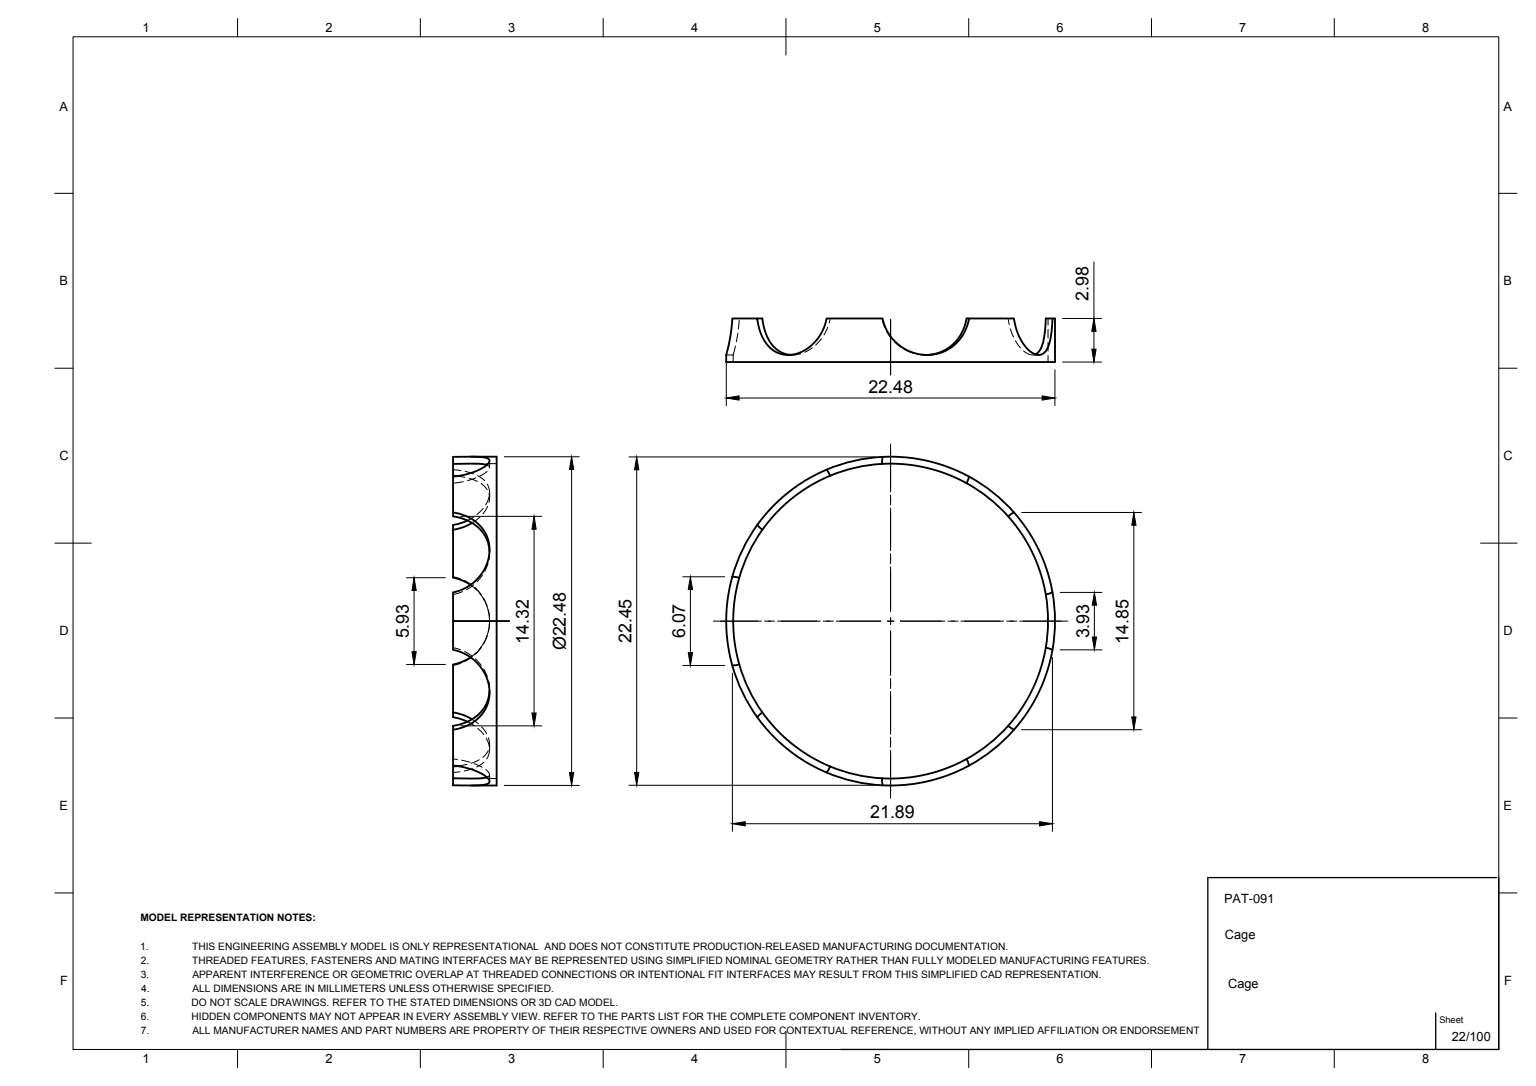
ISO-10303-21;
HEADER;
/* Generated by software containing ST-Developer
 * from STEP Tools, Inc. (www.steptools.com) 
 */

FILE_DESCRIPTION(
/* description */ ('PAT-091'),
/* implementation_level */ '2;1');

FILE_NAME(
/* name */ 'Cage.step',
/* time_stamp */ '2026-10-27T15:34:44-07:00',
/* author */ (''),
/* organization */ (''),
/* preprocessor_version */ 'ST-DEVELOPER v20.2',
/* originating_system */ 'Autodesk Translation Framework v15.17.0.0',
/* authorisation */ '');

FILE_SCHEMA (('AUTOMOTIVE_DESIGN { 1 0 10303 214 3 1 1 }'));
ENDSEC;

DATA;
#10=MECHANICAL_DESIGN_GEOMETRIC_PRESENTATION_REPRESENTATION('',(#1079,#1080,#1081,#1082,#1083,#1084,#1085),#25100);
#21=SPHERICAL_SURFACE('',#16189,0.321462);
#22=SPHERICAL_SURFACE('',#16202,0.321462);
#23=SPHERICAL_SURFACE('',#16203,0.321462);
#24=SPHERICAL_SURFACE('',#16216,0.321462);
#25=SPHERICAL_SURFACE('',#16217,0.321462);
#26=SPHERICAL_SURFACE('',#16230,0.321462);
#27=SPHERICAL_SURFACE('',#16231,0.321462);
#28=SPHERICAL_SURFACE('',#16244,0.321462);
#29=SPHERICAL_SURFACE('',#16245,0.321462);
#30=SPHERICAL_SURFACE('',#16258,0.321462);
#31=SPHERICAL_SURFACE('',#16259,0.321462);
#32=SPHERICAL_SURFACE('',#16272,0.321462);
#33=SPHERICAL_SURFACE('',#16280,0.321462);
#34=SPHERICAL_SURFACE('',#16286,0.321462);
#701=B_SPLINE_CURVE_WITH_KNOTS('',3,(#24299,#24300,#24301,#24302,#24303,
#24304),.UNSPECIFIED.,.F.,.F.,(4,2,4),(0.899240844561108,0.954818878854282,
0.98574345825674),.UNSPECIFIED.);
#702=B_SPLINE_CURVE_WITH_KNOTS('',3,(#24308,#24309,#24310,#24311,#24312,
#24313),.UNSPECIFIED.,.F.,.F.,(4,2,4),(1.23862523261148,1.28156721462942,
1.33421556357425),.UNSPECIFIED.);
#703=B_SPLINE_CURVE_WITH_KNOTS('',3,(#24324,#24325,#24326,#24327,#24328,
#24329),.UNSPECIFIED.,.F.,.F.,(4,2,4),(0.959827414101938,1.01247576304677,
1.05541774506471),.UNSPECIFIED.);
#704=B_SPLINE_CURVE_WITH_KNOTS('',3,(#24335,#24336,#24337,#24338,#24339,
#24340),.UNSPECIFIED.,.F.,.F.,(4,2,4),(1.13866312806976,1.16958770747221,
1.22516574176539),.UNSPECIFIED.);
#705=B_SPLINE_CURVE_WITH_KNOTS('',3,(#24347,#24348,#24349,#24350,#24351,
#24352),.UNSPECIFIED.,.F.,.F.,(4,2,4),(0.899240844561108,0.954818878854283,
0.985743458256741),.UNSPECIFIED.);
#706=B_SPLINE_CURVE_WITH_KNOTS('',3,(#24355,#24356,#24357,#24358,#24359,
#24360),.UNSPECIFIED.,.F.,.F.,(4,2,4),(1.23862523261148,1.28156721462942,
1.33421556357425),.UNSPECIFIED.);
#707=B_SPLINE_CURVE_WITH_KNOTS('',3,(#24369,#24370,#24371,#24372,#24373,
#24374),.UNSPECIFIED.,.F.,.F.,(4,2,4),(0.959827414101939,1.01247576304677,
1.05541774506471),.UNSPECIFIED.);
#708=B_SPLINE_CURVE_WITH_KNOTS('',3,(#24379,#24380,#24381,#24382,#24383,
#24384),.UNSPECIFIED.,.F.,.F.,(4,2,4),(1.13866312806975,1.16958770747221,
1.22516574176539),.UNSPECIFIED.);
#709=B_SPLINE_CURVE_WITH_KNOTS('',3,(#24391,#24392,#24393,#24394,#24395,
#24396),.UNSPECIFIED.,.F.,.F.,(4,2,4),(0.899240844561107,0.954818878854282,
0.98574345825674),.UNSPECIFIED.);
#710=B_SPLINE_CURVE_WITH_KNOTS('',3,(#24400,#24401,#24402,#24403,#24404,
#24405),.UNSPECIFIED.,.F.,.F.,(4,2,4),(1.23862523261148,1.28156721462942,
1.33421556357425),.UNSPECIFIED.);
#711=B_SPLINE_CURVE_WITH_KNOTS('',3,(#24411,#24412,#24413,#24414,#24415,
#24416),.UNSPECIFIED.,.F.,.F.,(4,2,4),(0.959827414101938,1.01247576304677,
1.05541774506471),.UNSPECIFIED.);
#712=B_SPLINE_CURVE_WITH_KNOTS('',3,(#24427,#24428,#24429,#24430,#24431,
#24432),.UNSPECIFIED.,.F.,.F.,(4,2,4),(1.13866312806976,1.16958770747221,
1.22516574176539),.UNSPECIFIED.);
#713=B_SPLINE_CURVE_WITH_KNOTS('',3,(#24439,#24440,#24441,#24442,#24443,
#24444),.UNSPECIFIED.,.F.,.F.,(4,2,4),(1.13866312806976,1.16958770747221,
1.22516574176539),.UNSPECIFIED.);
#714=B_SPLINE_CURVE_WITH_KNOTS('',3,(#24447,#24448,#24449,#24450,#24451,
#24452),.UNSPECIFIED.,.F.,.F.,(4,2,4),(0.959827414101938,1.01247576304677,
1.05541774506471),.UNSPECIFIED.);
#715=B_SPLINE_CURVE_WITH_KNOTS('',3,(#24457,#24458,#24459,#24460,#24461,
#24462),.UNSPECIFIED.,.F.,.F.,(4,2,4),(1.23862523261148,1.28156721462942,
1.33421556357425),.UNSPECIFIED.);
#716=B_SPLINE_CURVE_WITH_KNOTS('',3,(#24471,#24472,#24473,#24474,#24475,
#24476),.UNSPECIFIED.,.F.,.F.,(4,2,4),(0.899240844561108,0.954818878854282,
0.985743458256741),.UNSPECIFIED.);
#717=B_SPLINE_CURVE_WITH_KNOTS('',3,(#24483,#24484,#24485,#24486,#24487,
#24488),.UNSPECIFIED.,.F.,.F.,(4,2,4),(1.13866312806975,1.16958770747221,
1.22516574176539),.UNSPECIFIED.);
#718=B_SPLINE_CURVE_WITH_KNOTS('',3,(#24492,#24493,#24494,#24495,#24496,
#24497),.UNSPECIFIED.,.F.,.F.,(4,2,4),(0.959827414101939,1.01247576304677,
1.05541774506471),.UNSPECIFIED.);
#719=B_SPLINE_CURVE_WITH_KNOTS('',3,(#24502,#24503,#24504,#24505,#24506,
#24507),.UNSPECIFIED.,.F.,.F.,(4,2,4),(0.899240844561108,0.954818878854282,
0.985743458256741),.UNSPECIFIED.);
#720=B_SPLINE_CURVE_WITH_KNOTS('',3,(#24519,#24520,#24521,#24522,#24523,
#24524),.UNSPECIFIED.,.F.,.F.,(4,2,4),(1.23862523261148,1.28156721462942,
1.33421556357425),.UNSPECIFIED.);
#721=B_SPLINE_CURVE_WITH_KNOTS('',3,(#24529,#24530,#24531,#24532,#24533,
#24534),.UNSPECIFIED.,.F.,.F.,(4,2,4),(1.13866312806976,1.16958770747221,
1.22516574176539),.UNSPECIFIED.);
#722=B_SPLINE_CURVE_WITH_KNOTS('',3,(#24538,#24539,#24540,#24541,#24542,
#24543),.UNSPECIFIED.,.F.,.F.,(4,2,4),(0.959827414101938,1.01247576304677,
1.05541774506471),.UNSPECIFIED.);
#723=B_SPLINE_CURVE_WITH_KNOTS('',3,(#24548,#24549,#24550,#24551,#24552,
#24553),.UNSPECIFIED.,.F.,.F.,(4,2,4),(0.899240844561108,0.954818878854282,
0.98574345825674),.UNSPECIFIED.);
#724=B_SPLINE_CURVE_WITH_KNOTS('',3,(#24562,#24563,#24564,#24565,#24566,
#24567),.UNSPECIFIED.,.F.,.F.,(4,2,4),(1.23862523261148,1.28156721462942,
1.33421556357425),.UNSPECIFIED.);
#725=B_SPLINE_CURVE_WITH_KNOTS('',3,(#24575,#24576,#24577,#24578,#24579,
#24580),.UNSPECIFIED.,.F.,.F.,(4,2,4),(1.23862523261148,1.28156721462942,
1.33421556357425),.UNSPECIFIED.);
#726=B_SPLINE_CURVE_WITH_KNOTS('',3,(#24584,#24585,#24586,#24587,#24588,
#24589),.UNSPECIFIED.,.F.,.F.,(4,2,4),(0.959827414101938,1.01247576304677,
1.05541774506471),.UNSPECIFIED.);
#727=B_SPLINE_CURVE_WITH_KNOTS('',3,(#24600,#24601,#24602,#24603,#24604,
#24605),.UNSPECIFIED.,.F.,.F.,(4,2,4),(1.13866312806976,1.16958770747221,
1.22516574176539),.UNSPECIFIED.);
#728=B_SPLINE_CURVE_WITH_KNOTS('',3,(#24611,#24612,#24613,#24614,#24615,
#24616),.UNSPECIFIED.,.F.,.F.,(4,2,4),(0.899240844561108,0.954818878854282,
0.98574345825674),.UNSPECIFIED.);
#853=SHAPE_REPRESENTATION_RELATIONSHIP('SRR','None',#25621,#963);
#963=ADVANCED_BREP_SHAPE_REPRESENTATION('',(#1200,#1201,#1202,#1203,#1204,
#1205,#1206),#25091);
#1079=STYLED_ITEM('',(#26191),#1200);
#1080=STYLED_ITEM('',(#26191),#1201);
#1081=STYLED_ITEM('',(#26191),#1202);
#1082=STYLED_ITEM('',(#26191),#1203);
#1083=STYLED_ITEM('',(#26191),#1204);
#1084=STYLED_ITEM('',(#26191),#1205);
#1085=STYLED_ITEM('',(#26191),#1206);
#1200=MANIFOLD_SOLID_BREP('Body1',#13359);
#1201=MANIFOLD_SOLID_BREP('Body9',#13360);
#1202=MANIFOLD_SOLID_BREP('Body10',#13361);
#1203=MANIFOLD_SOLID_BREP('Body11',#13362);
#1204=MANIFOLD_SOLID_BREP('Body12',#13363);
#1205=MANIFOLD_SOLID_BREP('Body13',#13364);
#1206=MANIFOLD_SOLID_BREP('Body14',#13365);
#2028=PLANE('',#16192);
#2029=PLANE('',#16198);
#2030=PLANE('',#16206);
#2031=PLANE('',#16214);
#2032=PLANE('',#16223);
#2033=PLANE('',#16226);
#2034=PLANE('',#16237);
#2035=PLANE('',#16242);
#2036=PLANE('',#16251);
#2037=PLANE('',#16254);
#2038=PLANE('',#16265);
#2039=PLANE('',#16270);
#2040=PLANE('',#16276);
#2041=PLANE('',#16282);
#2798=FACE_OUTER_BOUND('',#4022,.T.);
#2799=FACE_OUTER_BOUND('',#4023,.T.);
#2800=FACE_OUTER_BOUND('',#4024,.T.);
#2801=FACE_OUTER_BOUND('',#4025,.T.);
#2802=FACE_OUTER_BOUND('',#4026,.T.);
#2803=FACE_OUTER_BOUND('',#4027,.T.);
#2804=FACE_OUTER_BOUND('',#4028,.T.);
#2805=FACE_OUTER_BOUND('',#4029,.T.);
#2806=FACE_OUTER_BOUND('',#4030,.T.);
#2807=FACE_OUTER_BOUND('',#4031,.T.);
#2808=FACE_OUTER_BOUND('',#4032,.T.);
#2809=FACE_OUTER_BOUND('',#4033,.T.);
#2810=FACE_OUTER_BOUND('',#4034,.T.);
#2811=FACE_OUTER_BOUND('',#4035,.T.);
#2812=FACE_OUTER_BOUND('',#4036,.T.);
#2813=FACE_OUTER_BOUND('',#4037,.T.);
#2814=FACE_OUTER_BOUND('',#4038,.T.);
#2815=FACE_OUTER_BOUND('',#4039,.T.);
#2816=FACE_OUTER_BOUND('',#4040,.T.);
#2817=FACE_OUTER_BOUND('',#4041,.T.);
#2818=FACE_OUTER_BOUND('',#4042,.T.);
#2819=FACE_OUTER_BOUND('',#4043,.T.);
#2820=FACE_OUTER_BOUND('',#4044,.T.);
#2821=FACE_OUTER_BOUND('',#4045,.T.);
#2822=FACE_OUTER_BOUND('',#4046,.T.);
#2823=FACE_OUTER_BOUND('',#4047,.T.);
#2824=FACE_OUTER_BOUND('',#4048,.T.);
#2825=FACE_OUTER_BOUND('',#4049,.T.);
#2826=FACE_OUTER_BOUND('',#4050,.T.);
#2827=FACE_OUTER_BOUND('',#4051,.T.);
#2828=FACE_OUTER_BOUND('',#4052,.T.);
#2829=FACE_OUTER_BOUND('',#4053,.T.);
#2830=FACE_OUTER_BOUND('',#4054,.T.);
#2831=FACE_OUTER_BOUND('',#4055,.T.);
#2832=FACE_OUTER_BOUND('',#4056,.T.);
#2833=FACE_OUTER_BOUND('',#4057,.T.);
#2834=FACE_OUTER_BOUND('',#4058,.T.);
#2835=FACE_OUTER_BOUND('',#4059,.T.);
#2836=FACE_OUTER_BOUND('',#4060,.T.);
#2837=FACE_OUTER_BOUND('',#4061,.T.);
#2838=FACE_OUTER_BOUND('',#4062,.T.);
#2839=FACE_OUTER_BOUND('',#4063,.T.);
#4022=EDGE_LOOP('',(#11786,#11787,#11788,#11789));
#4023=EDGE_LOOP('',(#11790,#11791,#11792,#11793));
#4024=EDGE_LOOP('',(#11794,#11795,#11796,#11797));
#4025=EDGE_LOOP('',(#11798,#11799,#11800,#11801));
#4026=EDGE_LOOP('',(#11802,#11803,#11804,#11805));
#4027=EDGE_LOOP('',(#11806,#11807,#11808,#11809));
#4028=EDGE_LOOP('',(#11810,#11811,#11812,#11813));
#4029=EDGE_LOOP('',(#11814,#11815,#11816,#11817));
#4030=EDGE_LOOP('',(#11818,#11819,#11820,#11821));
#4031=EDGE_LOOP('',(#11822,#11823,#11824,#11825));
#4032=EDGE_LOOP('',(#11826,#11827,#11828,#11829));
#4033=EDGE_LOOP('',(#11830,#11831,#11832,#11833));
#4034=EDGE_LOOP('',(#11834,#11835,#11836,#11837));
#4035=EDGE_LOOP('',(#11838,#11839,#11840,#11841));
#4036=EDGE_LOOP('',(#11842,#11843,#11844,#11845));
#4037=EDGE_LOOP('',(#11846,#11847,#11848,#11849));
#4038=EDGE_LOOP('',(#11850,#11851,#11852,#11853));
#4039=EDGE_LOOP('',(#11854,#11855,#11856,#11857));
#4040=EDGE_LOOP('',(#11858,#11859,#11860,#11861));
#4041=EDGE_LOOP('',(#11862,#11863,#11864,#11865));
#4042=EDGE_LOOP('',(#11866,#11867,#11868,#11869));
#4043=EDGE_LOOP('',(#11870,#11871,#11872,#11873));
#4044=EDGE_LOOP('',(#11874,#11875,#11876,#11877));
#4045=EDGE_LOOP('',(#11878,#11879,#11880,#11881));
#4046=EDGE_LOOP('',(#11882,#11883,#11884,#11885));
#4047=EDGE_LOOP('',(#11886,#11887,#11888,#11889));
#4048=EDGE_LOOP('',(#11890,#11891,#11892,#11893));
#4049=EDGE_LOOP('',(#11894,#11895,#11896,#11897));
#4050=EDGE_LOOP('',(#11898,#11899,#11900,#11901));
#4051=EDGE_LOOP('',(#11902,#11903,#11904,#11905));
#4052=EDGE_LOOP('',(#11906,#11907,#11908,#11909));
#4053=EDGE_LOOP('',(#11910,#11911,#11912,#11913));
#4054=EDGE_LOOP('',(#11914,#11915,#11916,#11917));
#4055=EDGE_LOOP('',(#11918,#11919,#11920,#11921));
#4056=EDGE_LOOP('',(#11922,#11923,#11924,#11925));
#4057=EDGE_LOOP('',(#11926,#11927,#11928,#11929));
#4058=EDGE_LOOP('',(#11930,#11931,#11932,#11933));
#4059=EDGE_LOOP('',(#11934,#11935,#11936,#11937));
#4060=EDGE_LOOP('',(#11938,#11939,#11940,#11941));
#4061=EDGE_LOOP('',(#11942,#11943,#11944,#11945));
#4062=EDGE_LOOP('',(#11946,#11947,#11948,#11949));
#4063=EDGE_LOOP('',(#11950,#11951,#11952,#11953));
#6287=CIRCLE('',#16190,0.267289037081583);
#6288=CIRCLE('',#16191,0.226018648221778);
#6289=CIRCLE('',#16193,1.308355);
#6290=CIRCLE('',#16194,0.226018648221778);
#6291=CIRCLE('',#16195,0.891645);
#6292=CIRCLE('',#16197,1.308355);
#6293=CIRCLE('',#16199,0.891645);
#6294=CIRCLE('',#16200,0.267289037081583);
#6295=CIRCLE('',#16204,0.226018648221778);
#6296=CIRCLE('',#16205,0.267289037081583);
#6297=CIRCLE('',#16207,0.891645);
#6298=CIRCLE('',#16208,0.267289037081583);
#6299=CIRCLE('',#16209,1.308355);
#6300=CIRCLE('',#16211,1.308355);
#6301=CIRCLE('',#16213,0.891645);
#6302=CIRCLE('',#16215,0.226018648221778);
#6303=CIRCLE('',#16218,0.267289037081583);
#6304=CIRCLE('',#16219,0.226018648221778);
#6305=CIRCLE('',#16221,1.308355);
#6306=CIRCLE('',#16222,1.308355);
#6307=CIRCLE('',#16224,0.226018648221778);
#6308=CIRCLE('',#16225,0.891645);
#6309=CIRCLE('',#16227,0.891645);
#6310=CIRCLE('',#16228,0.267289037081583);
#6311=CIRCLE('',#16232,0.267289037081583);
#6312=CIRCLE('',#16233,0.226018648221778);
#6313=CIRCLE('',#16235,1.308355);
#6314=CIRCLE('',#16236,1.308355);
#6315=CIRCLE('',#16238,0.891645);
#6316=CIRCLE('',#16239,0.226018648221778);
#6317=CIRCLE('',#16241,0.891645);
#6318=CIRCLE('',#16243,0.267289037081583);
#6319=CIRCLE('',#16246,0.226018648221778);
#6320=CIRCLE('',#16247,0.267289037081583);
#6321=CIRCLE('',#16249,0.891645);
#6322=CIRCLE('',#16250,0.891645);
#6323=CIRCLE('',#16252,0.267289037081583);
#6324=CIRCLE('',#16253,1.308355);
#6325=CIRCLE('',#16255,0.226018648221778);
#6326=CIRCLE('',#16256,1.308355);
#6327=CIRCLE('',#16260,0.226018648221778);
#6328=CIRCLE('',#16261,0.267289037081583);
#6329=CIRCLE('',#16263,0.891645);
#6330=CIRCLE('',#16264,0.891645);
#6331=CIRCLE('',#16266,0.267289037081583);
#6332=CIRCLE('',#16267,1.308355);
#6333=CIRCLE('',#16269,1.308355);
#6334=CIRCLE('',#16271,0.226018648221778);
#6335=CIRCLE('',#16274,1.308355);
#6336=CIRCLE('',#16275,1.308355);
#6337=CIRCLE('',#16277,0.226018648221778);
#6338=CIRCLE('',#16278,0.226018648221778);
#6339=CIRCLE('',#16279,0.891645);
#6340=CIRCLE('',#16281,0.267289037081583);
#6341=CIRCLE('',#16283,0.267289037081583);
#6342=CIRCLE('',#16284,0.891645);
#7325=VERTEX_POINT('',#24297);
#7326=VERTEX_POINT('',#24298);
#7327=VERTEX_POINT('',#24305);
#7328=VERTEX_POINT('',#24307);
#7329=VERTEX_POINT('',#24316);
#7330=VERTEX_POINT('',#24318);
#7331=VERTEX_POINT('',#24322);
#7332=VERTEX_POINT('',#24331);
#7333=VERTEX_POINT('',#24343);
#7334=VERTEX_POINT('',#24344);
#7335=VERTEX_POINT('',#24346);
#7336=VERTEX_POINT('',#24353);
#7337=VERTEX_POINT('',#24362);
#7338=VERTEX_POINT('',#24364);
#7339=VERTEX_POINT('',#24368);
#7340=VERTEX_POINT('',#24377);
#7341=VERTEX_POINT('',#24389);
#7342=VERTEX_POINT('',#24390);
#7343=VERTEX_POINT('',#24397);
#7344=VERTEX_POINT('',#24399);
#7345=VERTEX_POINT('',#24408);
#7346=VERTEX_POINT('',#24410);
#7347=VERTEX_POINT('',#24419);
#7348=VERTEX_POINT('',#24423);
#7349=VERTEX_POINT('',#24435);
#7350=VERTEX_POINT('',#24436);
#7351=VERTEX_POINT('',#24438);
#7352=VERTEX_POINT('',#24445);
#7353=VERTEX_POINT('',#24454);
#7354=VERTEX_POINT('',#24456);
#7355=VERTEX_POINT('',#24465);
#7356=VERTEX_POINT('',#24469);
#7357=VERTEX_POINT('',#24481);
#7358=VERTEX_POINT('',#24482);
#7359=VERTEX_POINT('',#24489);
#7360=VERTEX_POINT('',#24491);
#7361=VERTEX_POINT('',#24500);
#7362=VERTEX_POINT('',#24501);
#7363=VERTEX_POINT('',#24511);
#7364=VERTEX_POINT('',#24515);
#7365=VERTEX_POINT('',#24527);
#7366=VERTEX_POINT('',#24528);
#7367=VERTEX_POINT('',#24535);
#7368=VERTEX_POINT('',#24537);
#7369=VERTEX_POINT('',#24546);
#7370=VERTEX_POINT('',#24547);
#7371=VERTEX_POINT('',#24557);
#7372=VERTEX_POINT('',#24561);
#7373=VERTEX_POINT('',#24573);
#7374=VERTEX_POINT('',#24574);
#7375=VERTEX_POINT('',#24581);
#7376=VERTEX_POINT('',#24583);
#7377=VERTEX_POINT('',#24592);
#7378=VERTEX_POINT('',#24594);
#7379=VERTEX_POINT('',#24598);
#7380=VERTEX_POINT('',#24607);
#8828=EDGE_CURVE('',#7325,#7326,#701,.T.);
#8829=EDGE_CURVE('',#7327,#7325,#6287,.T.);
#8830=EDGE_CURVE('',#7328,#7327,#702,.T.);
#8831=EDGE_CURVE('',#7326,#7328,#6288,.T.);
#8832=EDGE_CURVE('',#7328,#7329,#6289,.T.);
#8833=EDGE_CURVE('',#7329,#7330,#6290,.T.);
#8834=EDGE_CURVE('',#7326,#7330,#6291,.T.);
#8835=EDGE_CURVE('',#7327,#7331,#6292,.T.);
#8836=EDGE_CURVE('',#7331,#7329,#703,.T.);
#8837=EDGE_CURVE('',#7325,#7332,#6293,.T.);
#8838=EDGE_CURVE('',#7332,#7331,#6294,.T.);
#8839=EDGE_CURVE('',#7330,#7332,#704,.T.);
#8840=EDGE_CURVE('',#7333,#7334,#6295,.T.);
#8841=EDGE_CURVE('',#7335,#7333,#705,.T.);
#8842=EDGE_CURVE('',#7336,#7335,#6296,.T.);
#8843=EDGE_CURVE('',#7334,#7336,#706,.T.);
#8844=EDGE_CURVE('',#7335,#7337,#6297,.T.);
#8845=EDGE_CURVE('',#7337,#7338,#6298,.T.);
#8846=EDGE_CURVE('',#7336,#7338,#6299,.T.);
#8847=EDGE_CURVE('',#7338,#7339,#707,.T.);
#8848=EDGE_CURVE('',#7334,#7339,#6300,.T.);
#8849=EDGE_CURVE('',#7333,#7340,#6301,.T.);
#8850=EDGE_CURVE('',#7340,#7337,#708,.T.);
#8851=EDGE_CURVE('',#7339,#7340,#6302,.T.);
#8852=EDGE_CURVE('',#7341,#7342,#709,.T.);
#8853=EDGE_CURVE('',#7343,#7341,#6303,.T.);
#8854=EDGE_CURVE('',#7344,#7343,#710,.T.);
#8855=EDGE_CURVE('',#7342,#7344,#6304,.T.);
#8856=EDGE_CURVE('',#7343,#7345,#6305,.T.);
#8857=EDGE_CURVE('',#7345,#7346,#711,.T.);
#8858=EDGE_CURVE('',#7344,#7346,#6306,.T.);
#8859=EDGE_CURVE('',#7346,#7347,#6307,.T.);
#8860=EDGE_CURVE('',#7342,#7347,#6308,.T.);
#8861=EDGE_CURVE('',#7341,#7348,#6309,.T.);
#8862=EDGE_CURVE('',#7348,#7345,#6310,.T.);
#8863=EDGE_CURVE('',#7347,#7348,#712,.T.);
#8864=EDGE_CURVE('',#7349,#7350,#6311,.T.);
#8865=EDGE_CURVE('',#7351,#7349,#713,.T.);
#8866=EDGE_CURVE('',#7352,#7351,#6312,.T.);
#8867=EDGE_CURVE('',#7350,#7352,#714,.T.);
#8868=EDGE_CURVE('',#7353,#7352,#6313,.T.);
#8869=EDGE_CURVE('',#7353,#7354,#715,.T.);
#8870=EDGE_CURVE('',#7354,#7350,#6314,.T.);
#8871=EDGE_CURVE('',#7355,#7351,#6315,.T.);
#8872=EDGE_CURVE('',#7355,#7353,#6316,.T.);
#8873=EDGE_CURVE('',#7356,#7349,#6317,.T.);
#8874=EDGE_CURVE('',#7356,#7355,#716,.T.);
#8875=EDGE_CURVE('',#7354,#7356,#6318,.T.);
#8876=EDGE_CURVE('',#7357,#7358,#717,.T.);
#8877=EDGE_CURVE('',#7359,#7357,#6319,.T.);
#8878=EDGE_CURVE('',#7360,#7359,#718,.T.);
#8879=EDGE_CURVE('',#7358,#7360,#6320,.T.);
#8880=EDGE_CURVE('',#7361,#7362,#719,.T.);
#8881=EDGE_CURVE('',#7362,#7357,#6321,.T.);
#8882=EDGE_CURVE('',#7361,#7358,#6322,.T.);
#8883=EDGE_CURVE('',#7363,#7361,#6323,.T.);
#8884=EDGE_CURVE('',#7363,#7360,#6324,.T.);
#8885=EDGE_CURVE('',#7362,#7364,#6325,.T.);
#8886=EDGE_CURVE('',#7364,#7359,#6326,.T.);
#8887=EDGE_CURVE('',#7364,#7363,#720,.T.);
#8888=EDGE_CURVE('',#7365,#7366,#721,.T.);
#8889=EDGE_CURVE('',#7367,#7365,#6327,.T.);
#8890=EDGE_CURVE('',#7368,#7367,#722,.T.);
#8891=EDGE_CURVE('',#7366,#7368,#6328,.T.);
#8892=EDGE_CURVE('',#7369,#7370,#723,.T.);
#8893=EDGE_CURVE('',#7370,#7365,#6329,.T.);
#8894=EDGE_CURVE('',#7369,#7366,#6330,.T.);
#8895=EDGE_CURVE('',#7371,#7369,#6331,.T.);
#8896=EDGE_CURVE('',#7371,#7368,#6332,.T.);
#8897=EDGE_CURVE('',#7372,#7371,#724,.T.);
#8898=EDGE_CURVE('',#7372,#7367,#6333,.T.);
#8899=EDGE_CURVE('',#7370,#7372,#6334,.T.);
#8900=EDGE_CURVE('',#7373,#7374,#725,.T.);
#8901=EDGE_CURVE('',#7374,#7375,#6335,.T.);
#8902=EDGE_CURVE('',#7375,#7376,#726,.T.);
#8903=EDGE_CURVE('',#7373,#7376,#6336,.T.);
#8904=EDGE_CURVE('',#7377,#7373,#6337,.T.);
#8905=EDGE_CURVE('',#7376,#7378,#6338,.T.);
#8906=EDGE_CURVE('',#7377,#7378,#6339,.T.);
#8907=EDGE_CURVE('',#7379,#7375,#6340,.T.);
#8908=EDGE_CURVE('',#7378,#7379,#727,.T.);
#8909=EDGE_CURVE('',#7374,#7380,#6341,.T.);
#8910=EDGE_CURVE('',#7380,#7379,#6342,.T.);
#8911=EDGE_CURVE('',#7380,#7377,#728,.T.);
#11786=ORIENTED_EDGE('',*,*,#8828,.F.);
#11787=ORIENTED_EDGE('',*,*,#8829,.F.);
#11788=ORIENTED_EDGE('',*,*,#8830,.F.);
#11789=ORIENTED_EDGE('',*,*,#8831,.F.);
#11790=ORIENTED_EDGE('',*,*,#8831,.T.);
#11791=ORIENTED_EDGE('',*,*,#8832,.T.);
#11792=ORIENTED_EDGE('',*,*,#8833,.T.);
#11793=ORIENTED_EDGE('',*,*,#8834,.F.);
#11794=ORIENTED_EDGE('',*,*,#8830,.T.);
#11795=ORIENTED_EDGE('',*,*,#8835,.T.);
#11796=ORIENTED_EDGE('',*,*,#8836,.T.);
#11797=ORIENTED_EDGE('',*,*,#8832,.F.);
#11798=ORIENTED_EDGE('',*,*,#8829,.T.);
#11799=ORIENTED_EDGE('',*,*,#8837,.T.);
#11800=ORIENTED_EDGE('',*,*,#8838,.T.);
#11801=ORIENTED_EDGE('',*,*,#8835,.F.);
#11802=ORIENTED_EDGE('',*,*,#8828,.T.);
#11803=ORIENTED_EDGE('',*,*,#8834,.T.);
#11804=ORIENTED_EDGE('',*,*,#8839,.T.);
#11805=ORIENTED_EDGE('',*,*,#8837,.F.);
#11806=ORIENTED_EDGE('',*,*,#8833,.F.);
#11807=ORIENTED_EDGE('',*,*,#8836,.F.);
#11808=ORIENTED_EDGE('',*,*,#8838,.F.);
#11809=ORIENTED_EDGE('',*,*,#8839,.F.);
#11810=ORIENTED_EDGE('',*,*,#8840,.F.);
#11811=ORIENTED_EDGE('',*,*,#8841,.F.);
#11812=ORIENTED_EDGE('',*,*,#8842,.F.);
#11813=ORIENTED_EDGE('',*,*,#8843,.F.);
#11814=ORIENTED_EDGE('',*,*,#8842,.T.);
#11815=ORIENTED_EDGE('',*,*,#8844,.T.);
#11816=ORIENTED_EDGE('',*,*,#8845,.T.);
#11817=ORIENTED_EDGE('',*,*,#8846,.F.);
#11818=ORIENTED_EDGE('',*,*,#8843,.T.);
#11819=ORIENTED_EDGE('',*,*,#8846,.T.);
#11820=ORIENTED_EDGE('',*,*,#8847,.T.);
#11821=ORIENTED_EDGE('',*,*,#8848,.F.);
#11822=ORIENTED_EDGE('',*,*,#8841,.T.);
#11823=ORIENTED_EDGE('',*,*,#8849,.T.);
#11824=ORIENTED_EDGE('',*,*,#8850,.T.);
#11825=ORIENTED_EDGE('',*,*,#8844,.F.);
#11826=ORIENTED_EDGE('',*,*,#8840,.T.);
#11827=ORIENTED_EDGE('',*,*,#8848,.T.);
#11828=ORIENTED_EDGE('',*,*,#8851,.T.);
#11829=ORIENTED_EDGE('',*,*,#8849,.F.);
#11830=ORIENTED_EDGE('',*,*,#8845,.F.);
#11831=ORIENTED_EDGE('',*,*,#8850,.F.);
#11832=ORIENTED_EDGE('',*,*,#8851,.F.);
#11833=ORIENTED_EDGE('',*,*,#8847,.F.);
#11834=ORIENTED_EDGE('',*,*,#8852,.F.);
#11835=ORIENTED_EDGE('',*,*,#8853,.F.);
#11836=ORIENTED_EDGE('',*,*,#8854,.F.);
#11837=ORIENTED_EDGE('',*,*,#8855,.F.);
#11838=ORIENTED_EDGE('',*,*,#8854,.T.);
#11839=ORIENTED_EDGE('',*,*,#8856,.T.);
#11840=ORIENTED_EDGE('',*,*,#8857,.T.);
#11841=ORIENTED_EDGE('',*,*,#8858,.F.);
#11842=ORIENTED_EDGE('',*,*,#8855,.T.);
#11843=ORIENTED_EDGE('',*,*,#8858,.T.);
#11844=ORIENTED_EDGE('',*,*,#8859,.T.);
#11845=ORIENTED_EDGE('',*,*,#8860,.F.);
#11846=ORIENTED_EDGE('',*,*,#8853,.T.);
#11847=ORIENTED_EDGE('',*,*,#8861,.T.);
#11848=ORIENTED_EDGE('',*,*,#8862,.T.);
#11849=ORIENTED_EDGE('',*,*,#8856,.F.);
#11850=ORIENTED_EDGE('',*,*,#8852,.T.);
#11851=ORIENTED_EDGE('',*,*,#8860,.T.);
#11852=ORIENTED_EDGE('',*,*,#8863,.T.);
#11853=ORIENTED_EDGE('',*,*,#8861,.F.);
#11854=ORIENTED_EDGE('',*,*,#8859,.F.);
#11855=ORIENTED_EDGE('',*,*,#8857,.F.);
#11856=ORIENTED_EDGE('',*,*,#8862,.F.);
#11857=ORIENTED_EDGE('',*,*,#8863,.F.);
#11858=ORIENTED_EDGE('',*,*,#8864,.F.);
#11859=ORIENTED_EDGE('',*,*,#8865,.F.);
#11860=ORIENTED_EDGE('',*,*,#8866,.F.);
#11861=ORIENTED_EDGE('',*,*,#8867,.F.);
#11862=ORIENTED_EDGE('',*,*,#8867,.T.);
#11863=ORIENTED_EDGE('',*,*,#8868,.F.);
#11864=ORIENTED_EDGE('',*,*,#8869,.T.);
#11865=ORIENTED_EDGE('',*,*,#8870,.T.);
#11866=ORIENTED_EDGE('',*,*,#8866,.T.);
#11867=ORIENTED_EDGE('',*,*,#8871,.F.);
#11868=ORIENTED_EDGE('',*,*,#8872,.T.);
#11869=ORIENTED_EDGE('',*,*,#8868,.T.);
#11870=ORIENTED_EDGE('',*,*,#8865,.T.);
#11871=ORIENTED_EDGE('',*,*,#8873,.F.);
#11872=ORIENTED_EDGE('',*,*,#8874,.T.);
#11873=ORIENTED_EDGE('',*,*,#8871,.T.);
#11874=ORIENTED_EDGE('',*,*,#8864,.T.);
#11875=ORIENTED_EDGE('',*,*,#8870,.F.);
#11876=ORIENTED_EDGE('',*,*,#8875,.T.);
#11877=ORIENTED_EDGE('',*,*,#8873,.T.);
#11878=ORIENTED_EDGE('',*,*,#8875,.F.);
#11879=ORIENTED_EDGE('',*,*,#8869,.F.);
#11880=ORIENTED_EDGE('',*,*,#8872,.F.);
#11881=ORIENTED_EDGE('',*,*,#8874,.F.);
#11882=ORIENTED_EDGE('',*,*,#8876,.F.);
#11883=ORIENTED_EDGE('',*,*,#8877,.F.);
#11884=ORIENTED_EDGE('',*,*,#8878,.F.);
#11885=ORIENTED_EDGE('',*,*,#8879,.F.);
#11886=ORIENTED_EDGE('',*,*,#8880,.T.);
#11887=ORIENTED_EDGE('',*,*,#8881,.T.);
#11888=ORIENTED_EDGE('',*,*,#8876,.T.);
#11889=ORIENTED_EDGE('',*,*,#8882,.F.);
#11890=ORIENTED_EDGE('',*,*,#8883,.T.);
#11891=ORIENTED_EDGE('',*,*,#8882,.T.);
#11892=ORIENTED_EDGE('',*,*,#8879,.T.);
#11893=ORIENTED_EDGE('',*,*,#8884,.F.);
#11894=ORIENTED_EDGE('',*,*,#8885,.T.);
#11895=ORIENTED_EDGE('',*,*,#8886,.T.);
#11896=ORIENTED_EDGE('',*,*,#8877,.T.);
#11897=ORIENTED_EDGE('',*,*,#8881,.F.);
#11898=ORIENTED_EDGE('',*,*,#8887,.T.);
#11899=ORIENTED_EDGE('',*,*,#8884,.T.);
#11900=ORIENTED_EDGE('',*,*,#8878,.T.);
#11901=ORIENTED_EDGE('',*,*,#8886,.F.);
#11902=ORIENTED_EDGE('',*,*,#8883,.F.);
#11903=ORIENTED_EDGE('',*,*,#8887,.F.);
#11904=ORIENTED_EDGE('',*,*,#8885,.F.);
#11905=ORIENTED_EDGE('',*,*,#8880,.F.);
#11906=ORIENTED_EDGE('',*,*,#8888,.F.);
#11907=ORIENTED_EDGE('',*,*,#8889,.F.);
#11908=ORIENTED_EDGE('',*,*,#8890,.F.);
#11909=ORIENTED_EDGE('',*,*,#8891,.F.);
#11910=ORIENTED_EDGE('',*,*,#8892,.T.);
#11911=ORIENTED_EDGE('',*,*,#8893,.T.);
#11912=ORIENTED_EDGE('',*,*,#8888,.T.);
#11913=ORIENTED_EDGE('',*,*,#8894,.F.);
#11914=ORIENTED_EDGE('',*,*,#8895,.T.);
#11915=ORIENTED_EDGE('',*,*,#8894,.T.);
#11916=ORIENTED_EDGE('',*,*,#8891,.T.);
#11917=ORIENTED_EDGE('',*,*,#8896,.F.);
#11918=ORIENTED_EDGE('',*,*,#8897,.T.);
#11919=ORIENTED_EDGE('',*,*,#8896,.T.);
#11920=ORIENTED_EDGE('',*,*,#8890,.T.);
#11921=ORIENTED_EDGE('',*,*,#8898,.F.);
#11922=ORIENTED_EDGE('',*,*,#8899,.T.);
#11923=ORIENTED_EDGE('',*,*,#8898,.T.);
#11924=ORIENTED_EDGE('',*,*,#8889,.T.);
#11925=ORIENTED_EDGE('',*,*,#8893,.F.);
#11926=ORIENTED_EDGE('',*,*,#8895,.F.);
#11927=ORIENTED_EDGE('',*,*,#8897,.F.);
#11928=ORIENTED_EDGE('',*,*,#8899,.F.);
#11929=ORIENTED_EDGE('',*,*,#8892,.F.);
#11930=ORIENTED_EDGE('',*,*,#8900,.T.);
#11931=ORIENTED_EDGE('',*,*,#8901,.T.);
#11932=ORIENTED_EDGE('',*,*,#8902,.T.);
#11933=ORIENTED_EDGE('',*,*,#8903,.F.);
#11934=ORIENTED_EDGE('',*,*,#8904,.T.);
#11935=ORIENTED_EDGE('',*,*,#8903,.T.);
#11936=ORIENTED_EDGE('',*,*,#8905,.T.);
#11937=ORIENTED_EDGE('',*,*,#8906,.F.);
#11938=ORIENTED_EDGE('',*,*,#8907,.F.);
#11939=ORIENTED_EDGE('',*,*,#8908,.F.);
#11940=ORIENTED_EDGE('',*,*,#8905,.F.);
#11941=ORIENTED_EDGE('',*,*,#8902,.F.);
#11942=ORIENTED_EDGE('',*,*,#8909,.T.);
#11943=ORIENTED_EDGE('',*,*,#8910,.T.);
#11944=ORIENTED_EDGE('',*,*,#8907,.T.);
#11945=ORIENTED_EDGE('',*,*,#8901,.F.);
#11946=ORIENTED_EDGE('',*,*,#8911,.T.);
#11947=ORIENTED_EDGE('',*,*,#8906,.T.);
#11948=ORIENTED_EDGE('',*,*,#8908,.T.);
#11949=ORIENTED_EDGE('',*,*,#8910,.F.);
#11950=ORIENTED_EDGE('',*,*,#8904,.F.);
#11951=ORIENTED_EDGE('',*,*,#8911,.F.);
#11952=ORIENTED_EDGE('',*,*,#8909,.F.);
#11953=ORIENTED_EDGE('',*,*,#8900,.F.);
#12396=CYLINDRICAL_SURFACE('',#16196,1.308355);
#12397=CYLINDRICAL_SURFACE('',#16201,0.891645);
#12398=CYLINDRICAL_SURFACE('',#16210,1.308355);
#12399=CYLINDRICAL_SURFACE('',#16212,0.891645);
#12400=CYLINDRICAL_SURFACE('',#16220,1.308355);
#12401=CYLINDRICAL_SURFACE('',#16229,0.891645);
#12402=CYLINDRICAL_SURFACE('',#16234,1.308355);
#12403=CYLINDRICAL_SURFACE('',#16240,0.891645);
#12404=CYLINDRICAL_SURFACE('',#16248,0.891645);
#12405=CYLINDRICAL_SURFACE('',#16257,1.308355);
#12406=CYLINDRICAL_SURFACE('',#16262,0.891645);
#12407=CYLINDRICAL_SURFACE('',#16268,1.308355);
#12408=CYLINDRICAL_SURFACE('',#16273,1.308355);
#12409=CYLINDRICAL_SURFACE('',#16285,0.891645);
#13165=ADVANCED_FACE('',(#2798),#21,.F.);
#13166=ADVANCED_FACE('',(#2799),#2028,.T.);
#13167=ADVANCED_FACE('',(#2800),#12396,.T.);
#13168=ADVANCED_FACE('',(#2801),#2029,.T.);
#13169=ADVANCED_FACE('',(#2802),#12397,.F.);
#13170=ADVANCED_FACE('',(#2803),#22,.F.);
#13171=ADVANCED_FACE('',(#2804),#23,.F.);
#13172=ADVANCED_FACE('',(#2805),#2030,.T.);
#13173=ADVANCED_FACE('',(#2806),#12398,.T.);
#13174=ADVANCED_FACE('',(#2807),#12399,.F.);
#13175=ADVANCED_FACE('',(#2808),#2031,.T.);
#13176=ADVANCED_FACE('',(#2809),#24,.F.);
#13177=ADVANCED_FACE('',(#2810),#25,.F.);
#13178=ADVANCED_FACE('',(#2811),#12400,.T.);
#13179=ADVANCED_FACE('',(#2812),#2032,.T.);
#13180=ADVANCED_FACE('',(#2813),#2033,.T.);
#13181=ADVANCED_FACE('',(#2814),#12401,.F.);
#13182=ADVANCED_FACE('',(#2815),#26,.F.);
#13183=ADVANCED_FACE('',(#2816),#27,.F.);
#13184=ADVANCED_FACE('',(#2817),#12402,.T.);
#13185=ADVANCED_FACE('',(#2818),#2034,.T.);
#13186=ADVANCED_FACE('',(#2819),#12403,.F.);
#13187=ADVANCED_FACE('',(#2820),#2035,.T.);
#13188=ADVANCED_FACE('',(#2821),#28,.F.);
#13189=ADVANCED_FACE('',(#2822),#29,.F.);
#13190=ADVANCED_FACE('',(#2823),#12404,.F.);
#13191=ADVANCED_FACE('',(#2824),#2036,.T.);
#13192=ADVANCED_FACE('',(#2825),#2037,.T.);
#13193=ADVANCED_FACE('',(#2826),#12405,.T.);
#13194=ADVANCED_FACE('',(#2827),#30,.F.);
#13195=ADVANCED_FACE('',(#2828),#31,.F.);
#13196=ADVANCED_FACE('',(#2829),#12406,.F.);
#13197=ADVANCED_FACE('',(#2830),#2038,.T.);
#13198=ADVANCED_FACE('',(#2831),#12407,.T.);
#13199=ADVANCED_FACE('',(#2832),#2039,.T.);
#13200=ADVANCED_FACE('',(#2833),#32,.F.);
#13201=ADVANCED_FACE('',(#2834),#12408,.T.);
#13202=ADVANCED_FACE('',(#2835),#2040,.T.);
#13203=ADVANCED_FACE('',(#2836),#33,.F.);
#13204=ADVANCED_FACE('',(#2837),#2041,.T.);
#13205=ADVANCED_FACE('',(#2838),#12409,.F.);
#13206=ADVANCED_FACE('',(#2839),#34,.F.);
#13359=CLOSED_SHELL('',(#13165,#13166,#13167,#13168,#13169,#13170));
#13360=CLOSED_SHELL('',(#13171,#13172,#13173,#13174,#13175,#13176));
#13361=CLOSED_SHELL('',(#13177,#13178,#13179,#13180,#13181,#13182));
#13362=CLOSED_SHELL('',(#13183,#13184,#13185,#13186,#13187,#13188));
#13363=CLOSED_SHELL('',(#13189,#13190,#13191,#13192,#13193,#13194));
#13364=CLOSED_SHELL('',(#13195,#13196,#13197,#13198,#13199,#13200));
#13365=CLOSED_SHELL('',(#13201,#13202,#13203,#13204,#13205,#13206));
#16188=AXIS2_PLACEMENT_3D('',#24295,#20394,#20395);
#16189=AXIS2_PLACEMENT_3D('',#24296,#20396,#20397);
#16190=AXIS2_PLACEMENT_3D('',#24306,#20398,#20399);
#16191=AXIS2_PLACEMENT_3D('',#24314,#20400,#20401);
#16192=AXIS2_PLACEMENT_3D('',#24315,#20402,#20403);
#16193=AXIS2_PLACEMENT_3D('',#24317,#20404,#20405);
#16194=AXIS2_PLACEMENT_3D('',#24319,#20406,#20407);
#16195=AXIS2_PLACEMENT_3D('',#24320,#20408,#20409);
#16196=AXIS2_PLACEMENT_3D('',#24321,#20410,#20411);
#16197=AXIS2_PLACEMENT_3D('',#24323,#20412,#20413);
#16198=AXIS2_PLACEMENT_3D('',#24330,#20414,#20415);
#16199=AXIS2_PLACEMENT_3D('',#24332,#20416,#20417);
#16200=AXIS2_PLACEMENT_3D('',#24333,#20418,#20419);
#16201=AXIS2_PLACEMENT_3D('',#24334,#20420,#20421);
#16202=AXIS2_PLACEMENT_3D('',#24341,#20422,#20423);
#16203=AXIS2_PLACEMENT_3D('',#24342,#20424,#20425);
#16204=AXIS2_PLACEMENT_3D('',#24345,#20426,#20427);
#16205=AXIS2_PLACEMENT_3D('',#24354,#20428,#20429);
#16206=AXIS2_PLACEMENT_3D('',#24361,#20430,#20431);
#16207=AXIS2_PLACEMENT_3D('',#24363,#20432,#20433);
#16208=AXIS2_PLACEMENT_3D('',#24365,#20434,#20435);
#16209=AXIS2_PLACEMENT_3D('',#24366,#20436,#20437);
#16210=AXIS2_PLACEMENT_3D('',#24367,#20438,#20439);
#16211=AXIS2_PLACEMENT_3D('',#24375,#20440,#20441);
#16212=AXIS2_PLACEMENT_3D('',#24376,#20442,#20443);
#16213=AXIS2_PLACEMENT_3D('',#24378,#20444,#20445);
#16214=AXIS2_PLACEMENT_3D('',#24385,#20446,#20447);
#16215=AXIS2_PLACEMENT_3D('',#24386,#20448,#20449);
#16216=AXIS2_PLACEMENT_3D('',#24387,#20450,#20451);
#16217=AXIS2_PLACEMENT_3D('',#24388,#20452,#20453);
#16218=AXIS2_PLACEMENT_3D('',#24398,#20454,#20455);
#16219=AXIS2_PLACEMENT_3D('',#24406,#20456,#20457);
#16220=AXIS2_PLACEMENT_3D('',#24407,#20458,#20459);
#16221=AXIS2_PLACEMENT_3D('',#24409,#20460,#20461);
#16222=AXIS2_PLACEMENT_3D('',#24417,#20462,#20463);
#16223=AXIS2_PLACEMENT_3D('',#24418,#20464,#20465);
#16224=AXIS2_PLACEMENT_3D('',#24420,#20466,#20467);
#16225=AXIS2_PLACEMENT_3D('',#24421,#20468,#20469);
#16226=AXIS2_PLACEMENT_3D('',#24422,#20470,#20471);
#16227=AXIS2_PLACEMENT_3D('',#24424,#20472,#20473);
#16228=AXIS2_PLACEMENT_3D('',#24425,#20474,#20475);
#16229=AXIS2_PLACEMENT_3D('',#24426,#20476,#20477);
#16230=AXIS2_PLACEMENT_3D('',#24433,#20478,#20479);
#16231=AXIS2_PLACEMENT_3D('',#24434,#20480,#20481);
#16232=AXIS2_PLACEMENT_3D('',#24437,#20482,#20483);
#16233=AXIS2_PLACEMENT_3D('',#24446,#20484,#20485);
#16234=AXIS2_PLACEMENT_3D('',#24453,#20486,#20487);
#16235=AXIS2_PLACEMENT_3D('',#24455,#20488,#20489);
#16236=AXIS2_PLACEMENT_3D('',#24463,#20490,#20491);
#16237=AXIS2_PLACEMENT_3D('',#24464,#20492,#20493);
#16238=AXIS2_PLACEMENT_3D('',#24466,#20494,#20495);
#16239=AXIS2_PLACEMENT_3D('',#24467,#20496,#20497);
#16240=AXIS2_PLACEMENT_3D('',#24468,#20498,#20499);
#16241=AXIS2_PLACEMENT_3D('',#24470,#20500,#20501);
#16242=AXIS2_PLACEMENT_3D('',#24477,#20502,#20503);
#16243=AXIS2_PLACEMENT_3D('',#24478,#20504,#20505);
#16244=AXIS2_PLACEMENT_3D('',#24479,#20506,#20507);
#16245=AXIS2_PLACEMENT_3D('',#24480,#20508,#20509);
#16246=AXIS2_PLACEMENT_3D('',#24490,#20510,#20511);
#16247=AXIS2_PLACEMENT_3D('',#24498,#20512,#20513);
#16248=AXIS2_PLACEMENT_3D('',#24499,#20514,#20515);
#16249=AXIS2_PLACEMENT_3D('',#24508,#20516,#20517);
#16250=AXIS2_PLACEMENT_3D('',#24509,#20518,#20519);
#16251=AXIS2_PLACEMENT_3D('',#24510,#20520,#20521);
#16252=AXIS2_PLACEMENT_3D('',#24512,#20522,#20523);
#16253=AXIS2_PLACEMENT_3D('',#24513,#20524,#20525);
#16254=AXIS2_PLACEMENT_3D('',#24514,#20526,#20527);
#16255=AXIS2_PLACEMENT_3D('',#24516,#20528,#20529);
#16256=AXIS2_PLACEMENT_3D('',#24517,#20530,#20531);
#16257=AXIS2_PLACEMENT_3D('',#24518,#20532,#20533);
#16258=AXIS2_PLACEMENT_3D('',#24525,#20534,#20535);
#16259=AXIS2_PLACEMENT_3D('',#24526,#20536,#20537);
#16260=AXIS2_PLACEMENT_3D('',#24536,#20538,#20539);
#16261=AXIS2_PLACEMENT_3D('',#24544,#20540,#20541);
#16262=AXIS2_PLACEMENT_3D('',#24545,#20542,#20543);
#16263=AXIS2_PLACEMENT_3D('',#24554,#20544,#20545);
#16264=AXIS2_PLACEMENT_3D('',#24555,#20546,#20547);
#16265=AXIS2_PLACEMENT_3D('',#24556,#20548,#20549);
#16266=AXIS2_PLACEMENT_3D('',#24558,#20550,#20551);
#16267=AXIS2_PLACEMENT_3D('',#24559,#20552,#20553);
#16268=AXIS2_PLACEMENT_3D('',#24560,#20554,#20555);
#16269=AXIS2_PLACEMENT_3D('',#24568,#20556,#20557);
#16270=AXIS2_PLACEMENT_3D('',#24569,#20558,#20559);
#16271=AXIS2_PLACEMENT_3D('',#24570,#20560,#20561);
#16272=AXIS2_PLACEMENT_3D('',#24571,#20562,#20563);
#16273=AXIS2_PLACEMENT_3D('',#24572,#20564,#20565);
#16274=AXIS2_PLACEMENT_3D('',#24582,#20566,#20567);
#16275=AXIS2_PLACEMENT_3D('',#24590,#20568,#20569);
#16276=AXIS2_PLACEMENT_3D('',#24591,#20570,#20571);
#16277=AXIS2_PLACEMENT_3D('',#24593,#20572,#20573);
#16278=AXIS2_PLACEMENT_3D('',#24595,#20574,#20575);
#16279=AXIS2_PLACEMENT_3D('',#24596,#20576,#20577);
#16280=AXIS2_PLACEMENT_3D('',#24597,#20578,#20579);
#16281=AXIS2_PLACEMENT_3D('',#24599,#20580,#20581);
#16282=AXIS2_PLACEMENT_3D('',#24606,#20582,#20583);
#16283=AXIS2_PLACEMENT_3D('',#24608,#20584,#20585);
#16284=AXIS2_PLACEMENT_3D('',#24609,#20586,#20587);
#16285=AXIS2_PLACEMENT_3D('',#24610,#20588,#20589);
#16286=AXIS2_PLACEMENT_3D('',#24617,#20590,#20591);
#20394=DIRECTION('axis',(0.,0.,1.));
#20395=DIRECTION('refdir',(1.,0.,0.));
#20396=DIRECTION('center_axis',(0.974927912181824,0.,-0.222520933956315));
#20397=DIRECTION('ref_axis',(-0.222520933956314,0.,-0.974927912181824));
#20398=DIRECTION('center_axis',(0.,-1.,0.));
#20399=DIRECTION('ref_axis',(0.,0.,-1.));
#20400=DIRECTION('center_axis',(0.,1.,0.));
#20401=DIRECTION('ref_axis',(0.,0.,1.));
#20402=DIRECTION('center_axis',(0.,-1.,0.));
#20403=DIRECTION('ref_axis',(0.,0.,-1.));
#20404=DIRECTION('center_axis',(0.,-1.,0.));
#20405=DIRECTION('ref_axis',(1.,0.,0.));
#20406=DIRECTION('center_axis',(0.,1.,0.));
#20407=DIRECTION('ref_axis',(0.,0.,1.));
#20408=DIRECTION('center_axis',(0.,-1.,0.));
#20409=DIRECTION('ref_axis',(1.,0.,0.));
#20410=DIRECTION('center_axis',(0.,-1.,0.));
#20411=DIRECTION('ref_axis',(1.,0.,0.));
#20412=DIRECTION('center_axis',(0.,-1.,0.));
#20413=DIRECTION('ref_axis',(1.,0.,0.));
#20414=DIRECTION('center_axis',(0.,1.,0.));
#20415=DIRECTION('ref_axis',(0.,0.,1.));
#20416=DIRECTION('center_axis',(0.,-1.,0.));
#20417=DIRECTION('ref_axis',(1.,0.,0.));
#20418=DIRECTION('center_axis',(0.,-1.,0.));
#20419=DIRECTION('ref_axis',(0.,0.,-1.));
#20420=DIRECTION('center_axis',(0.,-1.,0.));
#20421=DIRECTION('ref_axis',(1.,0.,0.));
#20422=DIRECTION('center_axis',(0.78183148246803,0.,0.623489801858734));
#20423=DIRECTION('ref_axis',(0.623489801858734,0.,-0.78183148246803));
#20424=DIRECTION('center_axis',(-0.433883739117558,0.,-0.900968867902419));
#20425=DIRECTION('ref_axis',(-0.900968867902419,0.,0.433883739117558));
#20426=DIRECTION('center_axis',(0.,1.,0.));
#20427=DIRECTION('ref_axis',(0.,0.,1.));
#20428=DIRECTION('center_axis',(0.,-1.,0.));
#20429=DIRECTION('ref_axis',(0.,0.,-1.));
#20430=DIRECTION('center_axis',(0.,1.,0.));
#20431=DIRECTION('ref_axis',(0.,0.,1.));
#20432=DIRECTION('center_axis',(0.,-1.,0.));
#20433=DIRECTION('ref_axis',(1.,0.,0.));
#20434=DIRECTION('center_axis',(0.,-1.,0.));
#20435=DIRECTION('ref_axis',(0.,0.,-1.));
#20436=DIRECTION('center_axis',(0.,-1.,0.));
#20437=DIRECTION('ref_axis',(1.,0.,0.));
#20438=DIRECTION('center_axis',(0.,-1.,0.));
#20439=DIRECTION('ref_axis',(-1.,0.,1.22464679914735E-16));
#20440=DIRECTION('center_axis',(0.,-1.,0.));
#20441=DIRECTION('ref_axis',(1.,0.,0.));
#20442=DIRECTION('center_axis',(0.,-1.,0.));
#20443=DIRECTION('ref_axis',(-1.,0.,1.22464679914735E-16));
#20444=DIRECTION('center_axis',(0.,-1.,0.));
#20445=DIRECTION('ref_axis',(1.,0.,0.));
#20446=DIRECTION('center_axis',(0.,-1.,0.));
#20447=DIRECTION('ref_axis',(0.,0.,-1.));
#20448=DIRECTION('center_axis',(0.,1.,0.));
#20449=DIRECTION('ref_axis',(0.,0.,1.));
#20450=DIRECTION('center_axis',(0.433883739117558,0.,-0.900968867902419));
#20451=DIRECTION('ref_axis',(-0.900968867902419,0.,-0.433883739117558));
#20452=DIRECTION('center_axis',(-0.974927912181824,0.,-0.222520933956315));
#20453=DIRECTION('ref_axis',(-0.222520933956315,0.,0.974927912181824));
#20454=DIRECTION('center_axis',(0.,-1.,0.));
#20455=DIRECTION('ref_axis',(0.,0.,-1.));
#20456=DIRECTION('center_axis',(0.,1.,0.));
#20457=DIRECTION('ref_axis',(0.,0.,1.));
#20458=DIRECTION('center_axis',(0.,-1.,0.));
#20459=DIRECTION('ref_axis',(1.,0.,0.));
#20460=DIRECTION('center_axis',(0.,-1.,0.));
#20461=DIRECTION('ref_axis',(1.,0.,0.));
#20462=DIRECTION('center_axis',(0.,-1.,0.));
#20463=DIRECTION('ref_axis',(1.,0.,0.));
#20464=DIRECTION('center_axis',(0.,-1.,0.));
#20465=DIRECTION('ref_axis',(0.,0.,-1.));
#20466=DIRECTION('center_axis',(0.,1.,0.));
#20467=DIRECTION('ref_axis',(0.,0.,1.));
#20468=DIRECTION('center_axis',(0.,-1.,0.));
#20469=DIRECTION('ref_axis',(1.,0.,0.));
#20470=DIRECTION('center_axis',(0.,1.,0.));
#20471=DIRECTION('ref_axis',(0.,0.,1.));
#20472=DIRECTION('center_axis',(0.,-1.,0.));
#20473=DIRECTION('ref_axis',(1.,0.,0.));
#20474=DIRECTION('center_axis',(0.,-1.,0.));
#20475=DIRECTION('ref_axis',(0.,0.,-1.));
#20476=DIRECTION('center_axis',(0.,-1.,0.));
#20477=DIRECTION('ref_axis',(1.,0.,0.));
#20478=DIRECTION('center_axis',(-0.433883739117558,0.,-0.900968867902419));
#20479=DIRECTION('ref_axis',(-0.900968867902419,0.,0.433883739117558));
#20480=DIRECTION('center_axis',(-0.78183148246803,0.,0.623489801858733));
#20481=DIRECTION('ref_axis',(0.623489801858733,0.,0.78183148246803));
#20482=DIRECTION('center_axis',(0.,-1.,0.));
#20483=DIRECTION('ref_axis',(0.,0.,-1.));
#20484=DIRECTION('center_axis',(0.,1.,0.));
#20485=DIRECTION('ref_axis',(0.,0.,1.));
#20486=DIRECTION('center_axis',(0.,-1.,0.));
#20487=DIRECTION('ref_axis',(1.,0.,0.));
#20488=DIRECTION('center_axis',(0.,-1.,0.));
#20489=DIRECTION('ref_axis',(1.,0.,0.));
#20490=DIRECTION('center_axis',(0.,-1.,0.));
#20491=DIRECTION('ref_axis',(1.,0.,0.));
#20492=DIRECTION('center_axis',(0.,-1.,0.));
#20493=DIRECTION('ref_axis',(0.,0.,-1.));
#20494=DIRECTION('center_axis',(0.,-1.,0.));
#20495=DIRECTION('ref_axis',(1.,0.,0.));
#20496=DIRECTION('center_axis',(0.,1.,0.));
#20497=DIRECTION('ref_axis',(0.,0.,1.));
#20498=DIRECTION('center_axis',(0.,-1.,0.));
#20499=DIRECTION('ref_axis',(1.,0.,0.));
#20500=DIRECTION('center_axis',(0.,-1.,0.));
#20501=DIRECTION('ref_axis',(1.,0.,0.));
#20502=DIRECTION('center_axis',(0.,1.,0.));
#20503=DIRECTION('ref_axis',(0.,0.,1.));
#20504=DIRECTION('center_axis',(0.,-1.,0.));
#20505=DIRECTION('ref_axis',(0.,0.,-1.));
#20506=DIRECTION('center_axis',(0.,0.,1.));
#20507=DIRECTION('ref_axis',(1.,0.,0.));
#20508=DIRECTION('center_axis',(-0.974927912181824,0.,-0.222520933956315));
#20509=DIRECTION('ref_axis',(-0.222520933956315,0.,0.974927912181824));
#20510=DIRECTION('center_axis',(0.,1.,0.));
#20511=DIRECTION('ref_axis',(0.,0.,1.));
#20512=DIRECTION('center_axis',(0.,-1.,0.));
#20513=DIRECTION('ref_axis',(0.,0.,-1.));
#20514=DIRECTION('center_axis',(0.,-1.,0.));
#20515=DIRECTION('ref_axis',(1.,0.,0.));
#20516=DIRECTION('center_axis',(0.,-1.,0.));
#20517=DIRECTION('ref_axis',(1.,0.,0.));
#20518=DIRECTION('center_axis',(0.,-1.,0.));
#20519=DIRECTION('ref_axis',(1.,0.,0.));
#20520=DIRECTION('center_axis',(0.,1.,0.));
#20521=DIRECTION('ref_axis',(0.,0.,1.));
#20522=DIRECTION('center_axis',(0.,-1.,0.));
#20523=DIRECTION('ref_axis',(0.,0.,-1.));
#20524=DIRECTION('center_axis',(0.,-1.,0.));
#20525=DIRECTION('ref_axis',(1.,0.,0.));
#20526=DIRECTION('center_axis',(0.,-1.,0.));
#20527=DIRECTION('ref_axis',(0.,0.,-1.));
#20528=DIRECTION('center_axis',(0.,1.,0.));
#20529=DIRECTION('ref_axis',(0.,0.,1.));
#20530=DIRECTION('center_axis',(0.,-1.,0.));
#20531=DIRECTION('ref_axis',(1.,0.,0.));
#20532=DIRECTION('center_axis',(0.,-1.,0.));
#20533=DIRECTION('ref_axis',(1.,0.,0.));
#20534=DIRECTION('center_axis',(-0.78183148246803,0.,0.623489801858733));
#20535=DIRECTION('ref_axis',(0.623489801858733,0.,0.78183148246803));
#20536=DIRECTION('center_axis',(0.974927912181824,0.,-0.222520933956315));
#20537=DIRECTION('ref_axis',(-0.222520933956314,0.,-0.974927912181824));
#20538=DIRECTION('center_axis',(0.,1.,0.));
#20539=DIRECTION('ref_axis',(0.,0.,1.));
#20540=DIRECTION('center_axis',(0.,-1.,0.));
#20541=DIRECTION('ref_axis',(0.,0.,-1.));
#20542=DIRECTION('center_axis',(0.,-1.,0.));
#20543=DIRECTION('ref_axis',(1.,0.,0.));
#20544=DIRECTION('center_axis',(0.,-1.,0.));
#20545=DIRECTION('ref_axis',(1.,0.,0.));
#20546=DIRECTION('center_axis',(0.,-1.,0.));
#20547=DIRECTION('ref_axis',(1.,0.,0.));
#20548=DIRECTION('center_axis',(0.,1.,0.));
#20549=DIRECTION('ref_axis',(0.,0.,1.));
#20550=DIRECTION('center_axis',(0.,-1.,0.));
#20551=DIRECTION('ref_axis',(0.,0.,-1.));
#20552=DIRECTION('center_axis',(0.,-1.,0.));
#20553=DIRECTION('ref_axis',(1.,0.,0.));
#20554=DIRECTION('center_axis',(0.,-1.,0.));
#20555=DIRECTION('ref_axis',(1.,0.,0.));
#20556=DIRECTION('center_axis',(0.,-1.,0.));
#20557=DIRECTION('ref_axis',(1.,0.,0.));
#20558=DIRECTION('center_axis',(0.,-1.,0.));
#20559=DIRECTION('ref_axis',(0.,0.,-1.));
#20560=DIRECTION('center_axis',(0.,1.,0.));
#20561=DIRECTION('ref_axis',(0.,0.,1.));
#20562=DIRECTION('center_axis',(0.433883739117558,0.,-0.900968867902419));
#20563=DIRECTION('ref_axis',(-0.900968867902419,0.,-0.433883739117558));
#20564=DIRECTION('center_axis',(0.,-1.,0.));
#20565=DIRECTION('ref_axis',(1.,0.,0.));
#20566=DIRECTION('center_axis',(0.,-1.,0.));
#20567=DIRECTION('ref_axis',(1.,0.,0.));
#20568=DIRECTION('center_axis',(0.,-1.,0.));
#20569=DIRECTION('ref_axis',(1.,0.,0.));
#20570=DIRECTION('center_axis',(0.,-1.,0.));
#20571=DIRECTION('ref_axis',(0.,0.,-1.));
#20572=DIRECTION('center_axis',(0.,1.,0.));
#20573=DIRECTION('ref_axis',(0.,0.,1.));
#20574=DIRECTION('center_axis',(0.,1.,0.));
#20575=DIRECTION('ref_axis',(0.,0.,1.));
#20576=DIRECTION('center_axis',(0.,-1.,0.));
#20577=DIRECTION('ref_axis',(1.,0.,0.));
#20578=DIRECTION('center_axis',(0.,0.,1.));
#20579=DIRECTION('ref_axis',(1.,0.,0.));
#20580=DIRECTION('center_axis',(0.,-1.,0.));
#20581=DIRECTION('ref_axis',(0.,0.,-1.));
#20582=DIRECTION('center_axis',(0.,1.,0.));
#20583=DIRECTION('ref_axis',(0.,0.,1.));
#20584=DIRECTION('center_axis',(0.,-1.,0.));
#20585=DIRECTION('ref_axis',(0.,0.,-1.));
#20586=DIRECTION('center_axis',(0.,-1.,0.));
#20587=DIRECTION('ref_axis',(1.,0.,0.));
#20588=DIRECTION('center_axis',(0.,-1.,0.));
#20589=DIRECTION('ref_axis',(1.,0.,0.));
#20590=DIRECTION('center_axis',(0.78183148246803,0.,0.623489801858734));
#20591=DIRECTION('ref_axis',(0.623489801858734,0.,-0.78183148246803));
#24295=CARTESIAN_POINT('',(0.,0.,0.));
#24296=CARTESIAN_POINT('Origin',(-0.244773027351946,0.,-1.07242070340001));
#24297=CARTESIAN_POINT('',(-0.0491413193775444,-0.17859,-0.890289804925809));
#24298=CARTESIAN_POINT('',(-0.120823405150736,-0.22859,-0.883420913717115));
#24299=CARTESIAN_POINT('Ctrl Pts',(-0.0491413193775443,-0.17859,-0.890289804925809));
#24300=CARTESIAN_POINT('Ctrl Pts',(-0.0622366108032282,-0.192197739766234,
-0.889566984227727));
#24301=CARTESIAN_POINT('Ctrl Pts',(-0.0768612314186783,-0.204076596372851,
-0.888465811801874));
#24302=CARTESIAN_POINT('Ctrl Pts',(-0.101256149639299,-0.219236411496476,
-0.885920360302595));
#24303=CARTESIAN_POINT('Ctrl Pts',(-0.110791504359706,-0.224284758603913,
-0.884792953245369));
#24304=CARTESIAN_POINT('Ctrl Pts',(-0.120823405150736,-0.22859,-0.883420913717114));
#24305=CARTESIAN_POINT('',(-0.110717377488918,-0.17859,-1.30366194557752));
#24306=CARTESIAN_POINT('Origin',(-0.244773027351946,-0.17859,-1.07242070340001));
#24307=CARTESIAN_POINT('',(-0.197287840980438,-0.22859,-1.29339487931037));
#24308=CARTESIAN_POINT('Ctrl Pts',(-0.197287840980438,-0.228590000000001,
-1.29339487931037));
#24309=CARTESIAN_POINT('Ctrl Pts',(-0.182957777157794,-0.223500193956903,
-1.2955807139676));
#24310=CARTESIAN_POINT('Ctrl Pts',(-0.169262868734191,-0.217292055674527,
-1.29742089529918));
#24311=CARTESIAN_POINT('Ctrl Pts',(-0.141475557257539,-0.202063936711524,
-1.30077481170484));
#24312=CARTESIAN_POINT('Ctrl Pts',(-0.12509796078425,-0.190965925779192,
-1.30244063166664));
#24313=CARTESIAN_POINT('Ctrl Pts',(-0.110717377488918,-0.178589999999999,
-1.30366194557752));
#24314=CARTESIAN_POINT('Origin',(-0.244773027351946,-0.22859,-1.07242070340001));
#24315=CARTESIAN_POINT('Origin',(0.891645,-0.22859,0.));
#24316=CARTESIAN_POINT('',(0.738933209129743,-0.22859,-1.07970853403602));
#24317=CARTESIAN_POINT('Origin',(0.,-0.22859,0.));
#24318=CARTESIAN_POINT('',(0.492160095813005,-0.22859,-0.743511429713312));
#24319=CARTESIAN_POINT('Origin',(0.685838782044607,-0.22859,-0.860014630714833));
#24320=CARTESIAN_POINT('Origin',(0.,-0.22859,0.));
#24321=CARTESIAN_POINT('Origin',(0.,-0.20359,0.));
#24322=CARTESIAN_POINT('',(0.665390629745762,-0.17859,-1.12652035750427));
#24323=CARTESIAN_POINT('Origin',(0.,-0.17859,0.));
#24324=CARTESIAN_POINT('Ctrl Pts',(0.665390629745762,-0.178589999999999,
-1.12652035750427));
#24325=CARTESIAN_POINT('Ctrl Pts',(0.677817179350845,-0.190965925779192,
-1.11918049044176));
#24326=CARTESIAN_POINT('Ctrl Pts',(0.691850111710621,-0.202063936711525,
-1.11057366572105));
#24327=CARTESIAN_POINT('Ctrl Pts',(0.715430404483016,-0.217292055674528,
-1.09549542885049));
#24328=CARTESIAN_POINT('Ctrl Pts',(0.726970665864658,-0.223500193956903,
-1.08789548468573));
#24329=CARTESIAN_POINT('Ctrl Pts',(0.738933209129742,-0.228590000000001,
-1.07970853403602));
#24330=CARTESIAN_POINT('Origin',(1.308355,-0.17859,0.));
#24331=CARTESIAN_POINT('',(0.430557068346269,-0.17859,-0.780801778252372));
#24332=CARTESIAN_POINT('Origin',(0.,-0.17859,0.));
#24333=CARTESIAN_POINT('Origin',(0.685838782044607,-0.17859,-0.860014630714833));
#24334=CARTESIAN_POINT('Origin',(0.,-0.20359,0.));
#24335=CARTESIAN_POINT('Ctrl Pts',(0.492160095813005,-0.22859,-0.743511429713312));
#24336=CARTESIAN_POINT('Ctrl Pts',(0.483716971155137,-0.224284758603913,
-0.74910027323947));
#24337=CARTESIAN_POINT('Ctrl Pts',(0.475615076997141,-0.219236411496476,
-0.754253267259386));
#24338=CARTESIAN_POINT('Ctrl Pts',(0.454740445159586,-0.204076596372851,
-0.767131198148022));
#24339=CARTESIAN_POINT('Ctrl Pts',(0.442041898089724,-0.192197739766234,
-0.774468705297715));
#24340=CARTESIAN_POINT('Ctrl Pts',(0.430557068346269,-0.17859,-0.780801778252372));
#24341=CARTESIAN_POINT('Origin',(0.685838782044607,0.,-0.860014630714833));
#24342=CARTESIAN_POINT('Origin',(-0.991065754692661,0.,0.477272113029314));
#24343=CARTESIAN_POINT('',(-0.834385970030061,-0.22859,0.314373756923179));
#24344=CARTESIAN_POINT('',(-1.21706609467953,-0.22859,0.480148859424376));
#24345=CARTESIAN_POINT('Origin',(-0.991065754692661,-0.22859,0.477272113029314));
#24346=CARTESIAN_POINT('',(-0.857033408469345,-0.17859,0.246017362786485));
#24347=CARTESIAN_POINT('Ctrl Pts',(-0.857033408469345,-0.17859,0.246017362786485));
#24348=CARTESIAN_POINT('Ctrl Pts',(-0.853414733916809,-0.192197739766234,
0.25862348517872));
#24349=CARTESIAN_POINT('Ctrl Pts',(-0.849086885944613,-0.204076596372852,
0.272636402105144));
#24350=CARTESIAN_POINT('Ctrl Pts',(-0.84117687424262,-0.219236411496476,
0.29585327254886));
#24351=CARTESIAN_POINT('Ctrl Pts',(-0.837955917596151,-0.224284758603913,
0.304898684347016));
#24352=CARTESIAN_POINT('Ctrl Pts',(-0.834385970030061,-0.22859,0.314373756923179));
#24353=CARTESIAN_POINT('',(-1.24633948454876,-0.17859,0.398033535370734));
#24354=CARTESIAN_POINT('Origin',(-0.991065754692661,-0.17859,0.477272113029314));
#24355=CARTESIAN_POINT('Ctrl Pts',(-1.21706609467953,-0.228590000000001,
0.480148859424375));
#24356=CARTESIAN_POINT('Ctrl Pts',(-1.22238586508374,-0.223500193956903,
0.466664474189734));
#24357=CARTESIAN_POINT('Ctrl Pts',(-1.22722731304024,-0.217292055674528,
0.453722404581342));
#24358=CARTESIAN_POINT('Ctrl Pts',(-1.23668039826116,-0.202063936711525,
0.427378095629262));
#24359=CARTESIAN_POINT('Ctrl Pts',(-1.24194881070179,-0.190965925779192,
0.411781799506707));
#24360=CARTESIAN_POINT('Ctrl Pts',(-1.24633948454876,-0.178589999999999,
0.398033535370735));
#24361=CARTESIAN_POINT('Origin',(1.308355,-0.17859,0.));
#24362=CARTESIAN_POINT('',(-0.857033408469345,-0.17859,-0.246017362786486));
#24363=CARTESIAN_POINT('Origin',(0.,-0.17859,0.));
#24364=CARTESIAN_POINT('',(-1.24633948454876,-0.17859,-0.398033535370734));
#24365=CARTESIAN_POINT('Origin',(-0.991065754692661,-0.17859,-0.477272113029314));
#24366=CARTESIAN_POINT('Origin',(0.,-0.17859,0.));
#24367=CARTESIAN_POINT('Origin',(0.,-0.20359,0.));
#24368=CARTESIAN_POINT('',(-1.21706609467953,-0.22859,-0.480148859424376));
#24369=CARTESIAN_POINT('Ctrl Pts',(-1.24633948454876,-0.178589999999999,
-0.398033535370735));
#24370=CARTESIAN_POINT('Ctrl Pts',(-1.24194881070179,-0.190965925779192,
-0.411781799506707));
#24371=CARTESIAN_POINT('Ctrl Pts',(-1.23668039826116,-0.202063936711525,
-0.427378095629262));
#24372=CARTESIAN_POINT('Ctrl Pts',(-1.22722731304024,-0.217292055674528,
-0.453722404581342));
#24373=CARTESIAN_POINT('Ctrl Pts',(-1.22238586508374,-0.223500193956903,
-0.466664474189735));
#24374=CARTESIAN_POINT('Ctrl Pts',(-1.21706609467953,-0.228590000000001,
-0.480148859424376));
#24375=CARTESIAN_POINT('Origin',(0.,-0.22859,0.));
#24376=CARTESIAN_POINT('Origin',(0.,-0.20359,0.));
#24377=CARTESIAN_POINT('',(-0.834385970030061,-0.22859,-0.314373756923179));
#24378=CARTESIAN_POINT('Origin',(0.,-0.22859,0.));
#24379=CARTESIAN_POINT('Ctrl Pts',(-0.834385970030061,-0.22859,-0.314373756923179));
#24380=CARTESIAN_POINT('Ctrl Pts',(-0.837955917596151,-0.224284758603913,
-0.304898684347017));
#24381=CARTESIAN_POINT('Ctrl Pts',(-0.84117687424262,-0.219236411496476,
-0.29585327254886));
#24382=CARTESIAN_POINT('Ctrl Pts',(-0.849086885944613,-0.204076596372851,
-0.272636402105144));
#24383=CARTESIAN_POINT('Ctrl Pts',(-0.853414733916809,-0.192197739766234,
-0.25862348517872));
#24384=CARTESIAN_POINT('Ctrl Pts',(-0.857033408469345,-0.17859,-0.246017362786486));
#24385=CARTESIAN_POINT('Origin',(0.891645,-0.22859,0.));
#24386=CARTESIAN_POINT('Origin',(-0.991065754692661,-0.22859,-0.477272113029314));
#24387=CARTESIAN_POINT('Origin',(-0.991065754692661,0.,-0.477272113029314));
#24388=CARTESIAN_POINT('Origin',(-0.244773027351946,0.,1.07242070340001));
#24389=CARTESIAN_POINT('',(-0.342007470572634,-0.17859,0.823445017045771));
#24390=CARTESIAN_POINT('',(-0.274443842703457,-0.22859,0.848358051312746));
#24391=CARTESIAN_POINT('Ctrl Pts',(-0.342007470572634,-0.17859,0.82344501704577));
#24392=CARTESIAN_POINT('Ctrl Pts',(-0.329895400534788,-0.192197739766234,
0.828475612108333));
#24393=CARTESIAN_POINT('Ctrl Pts',(-0.316241291845841,-0.204076596372851,
0.833828875110254));
#24394=CARTESIAN_POINT('Ctrl Pts',(-0.293157799979787,-0.219236411496476,
0.842120060887678));
#24395=CARTESIAN_POINT('Ctrl Pts',(-0.284077578642798,-0.224284758603913,
0.845241537587566));
#24396=CARTESIAN_POINT('Ctrl Pts',(-0.274443842703457,-0.22859,0.848358051312746));
#24397=CARTESIAN_POINT('',(-0.465884809239132,-0.17859,1.22259729696463));
#24398=CARTESIAN_POINT('Origin',(-0.244773027351946,-0.17859,1.07242070340001));
#24399=CARTESIAN_POINT('',(-0.383432803651627,-0.22859,1.25090850629007));
#24400=CARTESIAN_POINT('Ctrl Pts',(-0.383432803651627,-0.228590000000001,
1.25090850629007));
#24401=CARTESIAN_POINT('Ctrl Pts',(-0.397292143145055,-0.223500193956903,
1.24666029359345));
#24402=CARTESIAN_POINT('Ctrl Pts',(-0.410429254040296,-0.217292055674528,
1.2423762416108));
#24403=CARTESIAN_POINT('Ctrl Pts',(-0.436919966394242,-0.202063936711525,
1.23334155327433));
#24404=CARTESIAN_POINT('Ctrl Pts',(-0.45239844314147,-0.190965925779192,
1.22773643240386));
#24405=CARTESIAN_POINT('Ctrl Pts',(-0.465884809239131,-0.178589999999999,
1.22259729696463));
#24406=CARTESIAN_POINT('Origin',(-0.244773027351946,-0.22859,1.07242070340001));
#24407=CARTESIAN_POINT('Origin',(0.,-0.20359,0.));
#24408=CARTESIAN_POINT('',(-1.08827510730092,-0.17859,0.726257596761768));
#24409=CARTESIAN_POINT('Origin',(0.,-0.17859,0.));
#24410=CARTESIAN_POINT('',(-1.13422379278981,-0.22859,0.652172671839668));
#24411=CARTESIAN_POINT('Ctrl Pts',(-1.08827510730092,-0.178589999999999,
0.726257596761768));
#24412=CARTESIAN_POINT('Ctrl Pts',(-1.09628639266483,-0.190965925779192,
0.714252927236921));
#24413=CARTESIAN_POINT('Ctrl Pts',(-1.10519526655462,-0.202063936711525,
0.700409784949026));
#24414=CARTESIAN_POINT('Ctrl Pts',(-1.11989817444587,-0.217292055674528,
0.676593657348219));
#24415=CARTESIAN_POINT('Ctrl Pts',(-1.1269980984869,-0.223500193956903,
0.664739212499319));
#24416=CARTESIAN_POINT('Ctrl Pts',(-1.13422379278981,-0.228590000000001,
0.652172671839668));
#24417=CARTESIAN_POINT('Origin',(0.,-0.22859,0.));
#24418=CARTESIAN_POINT('Origin',(0.891645,-0.22859,0.));
#24419=CARTESIAN_POINT('',(-0.766018443552043,-0.22859,0.456340388485509));
#24420=CARTESIAN_POINT('Origin',(-0.991065754692661,-0.22859,0.477272113029314));
#24421=CARTESIAN_POINT('Origin',(0.,-0.22859,0.));
#24422=CARTESIAN_POINT('Origin',(1.308355,-0.17859,0.));
#24423=CARTESIAN_POINT('',(-0.7266957094931,-0.17859,0.516666383490662));
#24424=CARTESIAN_POINT('Origin',(0.,-0.17859,0.));
#24425=CARTESIAN_POINT('Origin',(-0.991065754692661,-0.17859,0.477272113029314));
#24426=CARTESIAN_POINT('Origin',(0.,-0.20359,0.));
#24427=CARTESIAN_POINT('Ctrl Pts',(-0.766018443552043,-0.22859,0.45634038848551));
#24428=CARTESIAN_POINT('Ctrl Pts',(-0.760836359413957,-0.224284758603913,
0.465039097006547));
#24429=CARTESIAN_POINT('Ctrl Pts',(-0.755772605319574,-0.219236411496476,
0.473197064326185));
#24430=CARTESIAN_POINT('Ctrl Pts',(-0.742552736711071,-0.204076596372852,
0.493856842454225));
#24431=CARTESIAN_POINT('Ctrl Pts',(-0.734295366171442,-0.192197739766234,
0.505977401048143));
#24432=CARTESIAN_POINT('Ctrl Pts',(-0.7266957094931,-0.17859,0.516666383490662));
#24433=CARTESIAN_POINT('Origin',(-0.991065754692661,0.,0.477272113029314));
#24434=CARTESIAN_POINT('Origin',(0.685838782044607,0.,0.860014630714833));
#24435=CARTESIAN_POINT('',(0.665417486529536,-0.17859,0.593506844649423));
#24436=CARTESIAN_POINT('',(0.950212795795148,-0.17859,0.899382259516035));
#24437=CARTESIAN_POINT('Origin',(0.685838782044607,-0.17859,0.860014630714833));
#24438=CARTESIAN_POINT('',(0.615354121677383,-0.22859,0.645267472417181));
#24439=CARTESIAN_POINT('Ctrl Pts',(0.615354121677383,-0.22859,0.64526747241718));
#24440=CARTESIAN_POINT('Ctrl Pts',(0.622681613212229,-0.224284758603913,
0.638279669203371));
#24441=CARTESIAN_POINT('Ctrl Pts',(0.629508251968404,-0.219236411496476,
0.631527555489181));
#24442=CARTESIAN_POINT('Ctrl Pts',(0.64670834881537,-0.204076596372851,
0.614041903462993));
#24443=CARTESIAN_POINT('Ctrl Pts',(0.656687581895314,-0.192197739766234,
0.60329448442429));
#24444=CARTESIAN_POINT('Ctrl Pts',(0.665417486529536,-0.17859,0.593506844649423));
#24445=CARTESIAN_POINT('',(0.888209879025751,-0.22859,0.960664362212974));
#24446=CARTESIAN_POINT('Origin',(0.685838782044607,-0.22859,0.860014630714833));
#24447=CARTESIAN_POINT('Ctrl Pts',(0.950212795795147,-0.178589999999999,
0.899382259516035));
#24448=CARTESIAN_POINT('Ctrl Pts',(0.940291787100225,-0.190965925779192,
0.909863975504277));
#24449=CARTESIAN_POINT('Ctrl Pts',(0.928778132229906,-0.202063936711525,
0.921629874276332));
#24450=CARTESIAN_POINT('Ctrl Pts',(0.90883082946763,-0.217292055674528,
0.941263736526708));
#24451=CARTESIAN_POINT('Ctrl Pts',(0.898853482029647,-0.223500193956903,
0.950823512787988));
#24452=CARTESIAN_POINT('Ctrl Pts',(0.888209879025751,-0.228590000000001,
0.960664362212974));
#24453=CARTESIAN_POINT('Origin',(0.,-0.20359,0.));
#24454=CARTESIAN_POINT('',(1.30486744394591,-0.22859,0.0954660136125388));
#24455=CARTESIAN_POINT('Origin',(0.,-0.22859,0.));
#24456=CARTESIAN_POINT('',(1.29561335303682,-0.17859,0.182150612015699));
#24457=CARTESIAN_POINT('Ctrl Pts',(1.30486744394591,-0.228590000000001,
0.0954660136125391));
#24458=CARTESIAN_POINT('Ctrl Pts',(1.30380973597919,-0.223500193956903,
0.109923186785982));
#24459=CARTESIAN_POINT('Ctrl Pts',(1.30255637630995,-0.217292055674527,
0.123684214131479));
#24460=CARTESIAN_POINT('Ctrl Pts',(1.29964294452704,-0.202063936711524,
0.151521156305556));
#24461=CARTESIAN_POINT('Ctrl Pts',(1.29762264084128,-0.190965925779192,
0.167858812055521));
#24462=CARTESIAN_POINT('Ctrl Pts',(1.29561335303682,-0.178589999999999,
0.182150612015698));
#24463=CARTESIAN_POINT('Origin',(0.,-0.17859,0.));
#24464=CARTESIAN_POINT('Origin',(0.891645,-0.22859,0.));
#24465=CARTESIAN_POINT('',(0.888157443945909,-0.22859,0.0787855366705671));
#24466=CARTESIAN_POINT('Origin',(0.,-0.22859,0.));
#24467=CARTESIAN_POINT('Origin',(1.1,-0.22859,0.));
#24468=CARTESIAN_POINT('Origin',(0.,-0.20359,0.));
#24469=CARTESIAN_POINT('',(0.878903353036818,-0.17859,0.150198874981266));
#24470=CARTESIAN_POINT('Origin',(0.,-0.17859,0.));
#24471=CARTESIAN_POINT('Ctrl Pts',(0.878903353036818,-0.17859,0.150198874981266));
#24472=CARTESIAN_POINT('Ctrl Pts',(0.881112631441229,-0.192197739766234,
0.137271067115392));
#24473=CARTESIAN_POINT('Ctrl Pts',(0.883293351945246,-0.204076596372851,
0.122768082355672));
#24474=CARTESIAN_POINT('Ctrl Pts',(0.886240100215735,-0.219236411496476,
0.0984183794220357));
#24475=CARTESIAN_POINT('Ctrl Pts',(0.887262775645244,-0.224284758603913,
0.0888712242812338));
#24476=CARTESIAN_POINT('Ctrl Pts',(0.888157443945909,-0.22859,0.0787855366705671));
#24477=CARTESIAN_POINT('Origin',(1.308355,-0.17859,0.));
#24478=CARTESIAN_POINT('Origin',(1.1,-0.17859,0.));
#24479=CARTESIAN_POINT('Origin',(1.1,0.,0.));
#24480=CARTESIAN_POINT('Origin',(-0.244773027351946,0.,1.07242070340001));
#24481=CARTESIAN_POINT('',(-0.120823405150736,-0.22859,0.883420913717115));
#24482=CARTESIAN_POINT('',(-0.0491413193775446,-0.17859,0.890289804925809));
#24483=CARTESIAN_POINT('Ctrl Pts',(-0.120823405150736,-0.22859,0.883420913717114));
#24484=CARTESIAN_POINT('Ctrl Pts',(-0.110791504359706,-0.224284758603913,
0.884792953245369));
#24485=CARTESIAN_POINT('Ctrl Pts',(-0.101256149639299,-0.219236411496475,
0.885920360302595));
#24486=CARTESIAN_POINT('Ctrl Pts',(-0.0768612314186785,-0.204076596372851,
0.888465811801873));
#24487=CARTESIAN_POINT('Ctrl Pts',(-0.0622366108032284,-0.192197739766234,
0.889566984227727));
#24488=CARTESIAN_POINT('Ctrl Pts',(-0.0491413193775446,-0.17859,0.890289804925809));
#24489=CARTESIAN_POINT('',(-0.197287840980439,-0.22859,1.29339487931037));
#24490=CARTESIAN_POINT('Origin',(-0.244773027351946,-0.22859,1.07242070340001));
#24491=CARTESIAN_POINT('',(-0.110717377488918,-0.17859,1.30366194557752));
#24492=CARTESIAN_POINT('Ctrl Pts',(-0.110717377488919,-0.178589999999999,
1.30366194557752));
#24493=CARTESIAN_POINT('Ctrl Pts',(-0.125097960784251,-0.190965925779192,
1.30244063166664));
#24494=CARTESIAN_POINT('Ctrl Pts',(-0.14147555725754,-0.202063936711525,
1.30077481170483));
#24495=CARTESIAN_POINT('Ctrl Pts',(-0.169262868734192,-0.217292055674528,
1.29742089529918));
#24496=CARTESIAN_POINT('Ctrl Pts',(-0.182957777157795,-0.223500193956903,
1.2955807139676));
#24497=CARTESIAN_POINT('Ctrl Pts',(-0.197287840980438,-0.228590000000001,
1.29339487931037));
#24498=CARTESIAN_POINT('Origin',(-0.244773027351946,-0.17859,1.07242070340001));
#24499=CARTESIAN_POINT('Origin',(0.,-0.20359,0.));
#24500=CARTESIAN_POINT('',(0.430557068346269,-0.17859,0.780801778252372));
#24501=CARTESIAN_POINT('',(0.492160095813005,-0.22859,0.743511429713312));
#24502=CARTESIAN_POINT('Ctrl Pts',(0.430557068346269,-0.17859,0.780801778252372));
#24503=CARTESIAN_POINT('Ctrl Pts',(0.442041898089724,-0.192197739766234,
0.774468705297715));
#24504=CARTESIAN_POINT('Ctrl Pts',(0.454740445159586,-0.204076596372851,
0.767131198148022));
#24505=CARTESIAN_POINT('Ctrl Pts',(0.475615076997141,-0.219236411496476,
0.754253267259386));
#24506=CARTESIAN_POINT('Ctrl Pts',(0.483716971155137,-0.224284758603913,
0.74910027323947));
#24507=CARTESIAN_POINT('Ctrl Pts',(0.492160095813005,-0.22859,0.743511429713312));
#24508=CARTESIAN_POINT('Origin',(0.,-0.22859,0.));
#24509=CARTESIAN_POINT('Origin',(0.,-0.17859,0.));
#24510=CARTESIAN_POINT('Origin',(1.308355,-0.17859,0.));
#24511=CARTESIAN_POINT('',(0.665390629745762,-0.17859,1.12652035750427));
#24512=CARTESIAN_POINT('Origin',(0.685838782044607,-0.17859,0.860014630714833));
#24513=CARTESIAN_POINT('Origin',(0.,-0.17859,0.));
#24514=CARTESIAN_POINT('Origin',(0.891645,-0.22859,0.));
#24515=CARTESIAN_POINT('',(0.738933209129742,-0.22859,1.07970853403602));
#24516=CARTESIAN_POINT('Origin',(0.685838782044607,-0.22859,0.860014630714833));
#24517=CARTESIAN_POINT('Origin',(0.,-0.22859,0.));
#24518=CARTESIAN_POINT('Origin',(0.,-0.20359,0.));
#24519=CARTESIAN_POINT('Ctrl Pts',(0.738933209129742,-0.228590000000001,
1.07970853403602));
#24520=CARTESIAN_POINT('Ctrl Pts',(0.726970665864657,-0.223500193956903,
1.08789548468573));
#24521=CARTESIAN_POINT('Ctrl Pts',(0.715430404483016,-0.217292055674527,
1.09549542885049));
#24522=CARTESIAN_POINT('Ctrl Pts',(0.69185011171062,-0.202063936711524,
1.11057366572105));
#24523=CARTESIAN_POINT('Ctrl Pts',(0.677817179350845,-0.190965925779192,
1.11918049044176));
#24524=CARTESIAN_POINT('Ctrl Pts',(0.665390629745762,-0.178589999999999,
1.12652035750427));
#24525=CARTESIAN_POINT('Origin',(0.685838782044607,0.,0.860014630714833));
#24526=CARTESIAN_POINT('Origin',(-0.244773027351946,0.,-1.07242070340001));
#24527=CARTESIAN_POINT('',(-0.274443842703457,-0.22859,-0.848358051312746));
#24528=CARTESIAN_POINT('',(-0.342007470572634,-0.17859,-0.823445017045771));
#24529=CARTESIAN_POINT('Ctrl Pts',(-0.274443842703457,-0.22859,-0.848358051312746));
#24530=CARTESIAN_POINT('Ctrl Pts',(-0.284077578642797,-0.224284758603913,
-0.845241537587567));
#24531=CARTESIAN_POINT('Ctrl Pts',(-0.293157799979787,-0.219236411496476,
-0.842120060887678));
#24532=CARTESIAN_POINT('Ctrl Pts',(-0.316241291845841,-0.204076596372851,
-0.833828875110254));
#24533=CARTESIAN_POINT('Ctrl Pts',(-0.329895400534788,-0.192197739766234,
-0.828475612108333));
#24534=CARTESIAN_POINT('Ctrl Pts',(-0.342007470572634,-0.17859,-0.82344501704577));
#24535=CARTESIAN_POINT('',(-0.383432803651626,-0.22859,-1.25090850629007));
#24536=CARTESIAN_POINT('Origin',(-0.244773027351946,-0.22859,-1.07242070340001));
#24537=CARTESIAN_POINT('',(-0.465884809239132,-0.17859,-1.22259729696463));
#24538=CARTESIAN_POINT('Ctrl Pts',(-0.465884809239131,-0.178589999999999,
-1.22259729696463));
#24539=CARTESIAN_POINT('Ctrl Pts',(-0.45239844314147,-0.190965925779192,
-1.22773643240386));
#24540=CARTESIAN_POINT('Ctrl Pts',(-0.436919966394242,-0.202063936711525,
-1.23334155327433));
#24541=CARTESIAN_POINT('Ctrl Pts',(-0.410429254040296,-0.217292055674528,
-1.2423762416108));
#24542=CARTESIAN_POINT('Ctrl Pts',(-0.397292143145055,-0.223500193956903,
-1.24666029359345));
#24543=CARTESIAN_POINT('Ctrl Pts',(-0.383432803651627,-0.228590000000001,
-1.25090850629007));
#24544=CARTESIAN_POINT('Origin',(-0.244773027351946,-0.17859,-1.07242070340001));
#24545=CARTESIAN_POINT('Origin',(0.,-0.20359,0.));
#24546=CARTESIAN_POINT('',(-0.7266957094931,-0.17859,-0.516666383490663));
#24547=CARTESIAN_POINT('',(-0.766018443552043,-0.22859,-0.45634038848551));
#24548=CARTESIAN_POINT('Ctrl Pts',(-0.7266957094931,-0.17859,-0.516666383490663));
#24549=CARTESIAN_POINT('Ctrl Pts',(-0.734295366171442,-0.192197739766234,
-0.505977401048143));
#24550=CARTESIAN_POINT('Ctrl Pts',(-0.74255273671107,-0.204076596372851,
-0.493856842454226));
#24551=CARTESIAN_POINT('Ctrl Pts',(-0.755772605319574,-0.219236411496476,
-0.473197064326185));
#24552=CARTESIAN_POINT('Ctrl Pts',(-0.760836359413957,-0.224284758603913,
-0.465039097006547));
#24553=CARTESIAN_POINT('Ctrl Pts',(-0.766018443552043,-0.22859,-0.45634038848551));
#24554=CARTESIAN_POINT('Origin',(0.,-0.22859,0.));
#24555=CARTESIAN_POINT('Origin',(0.,-0.17859,0.));
#24556=CARTESIAN_POINT('Origin',(1.308355,-0.17859,0.));
#24557=CARTESIAN_POINT('',(-1.08827510730092,-0.17859,-0.726257596761769));
#24558=CARTESIAN_POINT('Origin',(-0.991065754692661,-0.17859,-0.477272113029314));
#24559=CARTESIAN_POINT('Origin',(0.,-0.17859,0.));
#24560=CARTESIAN_POINT('Origin',(0.,-0.20359,0.));
#24561=CARTESIAN_POINT('',(-1.13422379278981,-0.22859,-0.652172671839668));
#24562=CARTESIAN_POINT('Ctrl Pts',(-1.13422379278981,-0.228590000000001,
-0.652172671839668));
#24563=CARTESIAN_POINT('Ctrl Pts',(-1.1269980984869,-0.223500193956903,
-0.66473921249932));
#24564=CARTESIAN_POINT('Ctrl Pts',(-1.11989817444587,-0.217292055674528,
-0.676593657348219));
#24565=CARTESIAN_POINT('Ctrl Pts',(-1.10519526655462,-0.202063936711525,
-0.700409784949027));
#24566=CARTESIAN_POINT('Ctrl Pts',(-1.09628639266483,-0.190965925779192,
-0.714252927236921));
#24567=CARTESIAN_POINT('Ctrl Pts',(-1.08827510730092,-0.178589999999999,
-0.726257596761768));
#24568=CARTESIAN_POINT('Origin',(0.,-0.22859,0.));
#24569=CARTESIAN_POINT('Origin',(0.891645,-0.22859,0.));
#24570=CARTESIAN_POINT('Origin',(-0.991065754692661,-0.22859,-0.477272113029314));
#24571=CARTESIAN_POINT('Origin',(-0.991065754692661,0.,-0.477272113029314));
#24572=CARTESIAN_POINT('Origin',(0.,-0.20359,0.));
#24573=CARTESIAN_POINT('',(0.888209879025751,-0.22859,-0.960664362212974));
#24574=CARTESIAN_POINT('',(0.950212795795148,-0.17859,-0.899382259516035));
#24575=CARTESIAN_POINT('Ctrl Pts',(0.888209879025752,-0.228590000000001,
-0.960664362212974));
#24576=CARTESIAN_POINT('Ctrl Pts',(0.898853482029647,-0.223500193956903,
-0.950823512787987));
#24577=CARTESIAN_POINT('Ctrl Pts',(0.908830829467631,-0.217292055674528,
-0.941263736526708));
#24578=CARTESIAN_POINT('Ctrl Pts',(0.928778132229906,-0.202063936711525,
-0.921629874276332));
#24579=CARTESIAN_POINT('Ctrl Pts',(0.940291787100225,-0.190965925779191,
-0.909863975504277));
#24580=CARTESIAN_POINT('Ctrl Pts',(0.950212795795148,-0.178589999999999,
-0.899382259516035));
#24581=CARTESIAN_POINT('',(1.29561335303682,-0.17859,-0.182150612015699));
#24582=CARTESIAN_POINT('Origin',(0.,-0.17859,0.));
#24583=CARTESIAN_POINT('',(1.30486744394591,-0.22859,-0.0954660136125388));
#24584=CARTESIAN_POINT('Ctrl Pts',(1.29561335303682,-0.178589999999999,
-0.182150612015698));
#24585=CARTESIAN_POINT('Ctrl Pts',(1.29762264084128,-0.190965925779192,
-0.167858812055521));
#24586=CARTESIAN_POINT('Ctrl Pts',(1.29964294452704,-0.202063936711524,
-0.151521156305556));
#24587=CARTESIAN_POINT('Ctrl Pts',(1.30255637630995,-0.217292055674527,
-0.123684214131479));
#24588=CARTESIAN_POINT('Ctrl Pts',(1.30380973597919,-0.223500193956903,
-0.109923186785982));
#24589=CARTESIAN_POINT('Ctrl Pts',(1.30486744394591,-0.228590000000001,
-0.0954660136125391));
#24590=CARTESIAN_POINT('Origin',(0.,-0.22859,0.));
#24591=CARTESIAN_POINT('Origin',(0.891645,-0.22859,0.));
#24592=CARTESIAN_POINT('',(0.615354121677383,-0.22859,-0.64526747241718));
#24593=CARTESIAN_POINT('Origin',(0.685838782044607,-0.22859,-0.860014630714833));
#24594=CARTESIAN_POINT('',(0.888157443945909,-0.22859,-0.0787855366705671));
#24595=CARTESIAN_POINT('Origin',(1.1,-0.22859,0.));
#24596=CARTESIAN_POINT('Origin',(0.,-0.22859,0.));
#24597=CARTESIAN_POINT('Origin',(1.1,0.,0.));
#24598=CARTESIAN_POINT('',(0.878903353036818,-0.17859,-0.150198874981266));
#24599=CARTESIAN_POINT('Origin',(1.1,-0.17859,0.));
#24600=CARTESIAN_POINT('Ctrl Pts',(0.888157443945909,-0.22859,-0.0787855366705672));
#24601=CARTESIAN_POINT('Ctrl Pts',(0.887262775645244,-0.224284758603913,
-0.0888712242812339));
#24602=CARTESIAN_POINT('Ctrl Pts',(0.886240100215735,-0.219236411496476,
-0.0984183794220357));
#24603=CARTESIAN_POINT('Ctrl Pts',(0.883293351945246,-0.204076596372851,
-0.122768082355672));
#24604=CARTESIAN_POINT('Ctrl Pts',(0.881112631441229,-0.192197739766234,
-0.137271067115392));
#24605=CARTESIAN_POINT('Ctrl Pts',(0.878903353036818,-0.17859,-0.150198874981266));
#24606=CARTESIAN_POINT('Origin',(1.308355,-0.17859,0.));
#24607=CARTESIAN_POINT('',(0.665417486529536,-0.17859,-0.593506844649423));
#24608=CARTESIAN_POINT('Origin',(0.685838782044607,-0.17859,-0.860014630714833));
#24609=CARTESIAN_POINT('Origin',(0.,-0.17859,0.));
#24610=CARTESIAN_POINT('Origin',(0.,-0.20359,0.));
#24611=CARTESIAN_POINT('Ctrl Pts',(0.665417486529536,-0.17859,-0.593506844649423));
#24612=CARTESIAN_POINT('Ctrl Pts',(0.656687581895314,-0.192197739766234,
-0.60329448442429));
#24613=CARTESIAN_POINT('Ctrl Pts',(0.64670834881537,-0.204076596372851,
-0.614041903462993));
#24614=CARTESIAN_POINT('Ctrl Pts',(0.629508251968404,-0.219236411496476,
-0.63152755548918));
#24615=CARTESIAN_POINT('Ctrl Pts',(0.622681613212229,-0.224284758603913,
-0.638279669203371));
#24616=CARTESIAN_POINT('Ctrl Pts',(0.615354121677383,-0.22859,-0.64526747241718));
#24617=CARTESIAN_POINT('Origin',(0.685838782044607,0.,-0.860014630714833));
#24970=UNCERTAINTY_MEASURE_WITH_UNIT(LENGTH_MEASURE(0.001),#25101,
'DISTANCE_ACCURACY_VALUE',
'Maximum model space distance between geometric entities at asserted c
onnectivities');
#24979=UNCERTAINTY_MEASURE_WITH_UNIT(LENGTH_MEASURE(0.001),#25101,
'DISTANCE_ACCURACY_VALUE',
'Maximum model space distance between geometric entities at asserted c
onnectivities');
#25091=(
GEOMETRIC_REPRESENTATION_CONTEXT(3)
GLOBAL_UNCERTAINTY_ASSIGNED_CONTEXT((#24970))
GLOBAL_UNIT_ASSIGNED_CONTEXT((#25101,#25103,#25104))
REPRESENTATION_CONTEXT('','3D')
);
#25100=(
GEOMETRIC_REPRESENTATION_CONTEXT(3)
GLOBAL_UNCERTAINTY_ASSIGNED_CONTEXT((#24979))
GLOBAL_UNIT_ASSIGNED_CONTEXT((#25101,#25103,#25104))
REPRESENTATION_CONTEXT('','3D')
);
#25101=(
LENGTH_UNIT()
NAMED_UNIT(*)
SI_UNIT(.CENTI.,.METRE.)
);
#25103=(
NAMED_UNIT(*)
PLANE_ANGLE_UNIT()
SI_UNIT($,.RADIAN.)
);
#25104=(
NAMED_UNIT(*)
SI_UNIT($,.STERADIAN.)
SOLID_ANGLE_UNIT()
);
#25216=SHAPE_DEFINITION_REPRESENTATION(#25410,#25621);
#25410=PRODUCT_DEFINITION_SHAPE('',$,#25742);
#25621=SHAPE_REPRESENTATION('',(#16188),#25091);
#25630=PRODUCT_DEFINITION_CONTEXT('part definition',#25992,'design');
#25742=PRODUCT_DEFINITION('Cage','Cage',#25862,#25630);
#25862=PRODUCT_DEFINITION_FORMATION('',$,#26105);
#25992=APPLICATION_CONTEXT(
'Core Data for Automotive Mechanical Design Process');
#25993=PRODUCT_CONTEXT('part definition',#25992,'mechanical');
#26105=PRODUCT('Cage','Cage','Cage',(#25993));
#26185=COLOUR_RGB('Grey',0.48,0.52,0.57);
#26186=FILL_AREA_STYLE_COLOUR('',#26185);
#26187=FILL_AREA_STYLE('',(#26186));
#26188=SURFACE_STYLE_FILL_AREA(#26187);
#26189=SURFACE_SIDE_STYLE('',(#26188));
#26190=SURFACE_STYLE_USAGE(.BOTH.,#26189);
#26191=PRESENTATION_STYLE_ASSIGNMENT((#26190));
ENDSEC;
END-ISO-10303-21;
